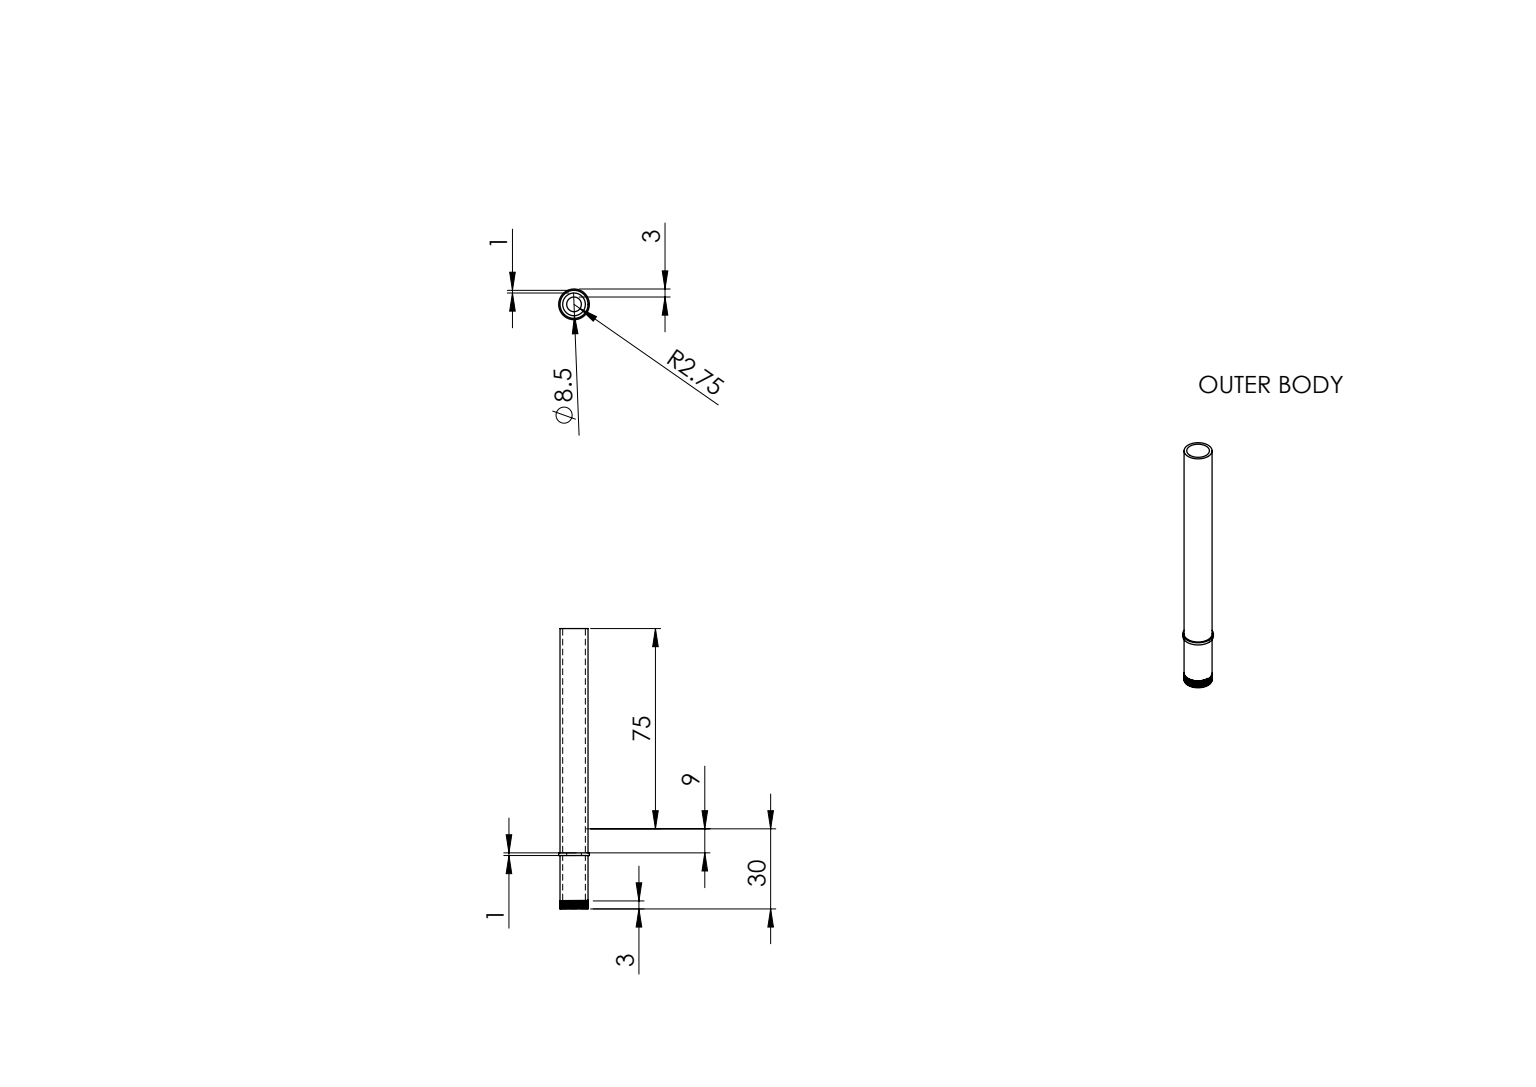
ISO-10303-21;
HEADER;
FILE_DESCRIPTION (('STEP AP214'),
    '1' );
FILE_NAME ('outer body.step',
    '2026-10-27T10:49:47',
    ( '' ),
    ( '' ),
    'SwSTEP 2.0',
    'SolidWorks 2026',
    '' );
FILE_SCHEMA (( 'AUTOMOTIVE_DESIGN' ));
ENDSEC;

DATA;
#4=CARTESIAN_POINT ( 'NONE',  ( 5.114683531250000748, -27.33854166700806587, -2.952963913586932776 ) ) ;
#6=CARTESIAN_POINT ( 'NONE',  ( 5.250000000000000000, -29.22916666666666430, -3.031088913245534755 ) ) ;
#8=ADVANCED_FACE ( 'NONE', ( #6134 ), #1014, .T. ) ;
#9=CARTESIAN_POINT ( 'NONE',  ( 5.114683531250000748, -28.90104166700806587, -2.952963913586932776 ) ) ;
#12=CARTESIAN_POINT ( 'NONE',  ( -5.114683531249999859, -28.31770833367473372, -2.952963913586935440 ) ) ;
#16=DIRECTION ( 'NONE',  ( 1.000000000000000000, 0.000000000000000000, -0.000000000000000000 ) ) ;
#17=CARTESIAN_POINT ( 'NONE',  ( -5.114683531249999859, -29.56770833367473017, -2.952963913586935440 ) ) ;
#19=EDGE_LOOP ( 'NONE', ( #3750, #4304, #1709, #1694 ) ) ;
#21=CARTESIAN_POINT ( 'NONE',  ( 2.557341765624996821, -29.15104166700806587, 4.429445870380401828 ) ) ;
#23=ORIENTED_EDGE ( 'NONE', *, *, #2711, .F. ) ;
#32=CARTESIAN_POINT ( 'NONE',  ( -5.114683531249999859, -28.75520833367473017, -2.952963913586935440 ) ) ;
#37=( BOUNDED_CURVE ( )  B_SPLINE_CURVE ( 2, ( #980, #8007, #3923, #3739, #4569, #5213, #3046, #6700, #6561 ),
 .UNSPECIFIED., .F., .F. ) 
 B_SPLINE_CURVE_WITH_KNOTS ( ( 3, 2, 2, 2, 3 ),
 ( 0.1041666666666666713, 0.1111111111111111049, 0.1250000000000000000, 0.1388888888888888951, 0.1458333333333333426 ),
 .UNSPECIFIED. ) 
 CURVE ( )  GEOMETRIC_REPRESENTATION_ITEM ( )  RATIONAL_B_SPLINE_CURVE ( ( 0.9330127018922194093, 0.9330127018922194093, 1.000000000000000000, 0.8660254037844387076, 1.000000000000000000, 0.8660254037844387076, 1.000000000000000000, 0.9330127018922194093, 0.9330127018922194093 ) ) 
 REPRESENTATION_ITEM ( '' )  );
#41=VECTOR ( 'NONE', #4397, 1000.000000000000000 ) ;
#44=CARTESIAN_POINT ( 'NONE',  ( 2.033577675846918216E-14, -27.81249999999999645, 5.250000000000000888 ) ) ;
#45=ORIENTED_EDGE ( 'NONE', *, *, #6013, .T. ) ;
#52=CARTESIAN_POINT ( 'NONE',  ( -2.624999999999998668, -28.91666666666666785, -4.546633369868303021 ) ) ;
#55=CARTESIAN_POINT ( 'NONE',  ( 5.114683531250000748, -28.42187500034139802, 0.000000000000000000 ) ) ;
#56=CARTESIAN_POINT ( 'NONE',  ( 3.616337804771879580E-16, -28.35937500034139447, -5.905927827173866440 ) ) ;
#65=CARTESIAN_POINT ( 'NONE',  ( 5.250000000000000000, -27.03125000068279604, 0.000000000000000000 ) ) ;
#74=EDGE_CURVE ( 'NONE', #2716, #8116, #2372, .T. ) ;
#76=CARTESIAN_POINT ( 'NONE',  ( -2.557341765624999042, -27.02604166700806232, -4.429445870380400052 ) ) ;
#79=EDGE_CURVE ( 'NONE', #7374, #1200, #6541, .T. ) ;
#83=FACE_OUTER_BOUND ( 'NONE', #879, .T. ) ;
#84=CARTESIAN_POINT ( 'NONE',  ( 0.000000000000000000, -30.00000000000000000, 0.000000000000000000 ) ) ;
#88=EDGE_LOOP ( 'NONE', ( #8020, #7590 ) ) ;
#91=ORIENTED_EDGE ( 'NONE', *, *, #709, .F. ) ;
#92=CARTESIAN_POINT ( 'NONE',  ( -2.625000000000002220, -28.58333333333333215, 4.546633369868302132 ) ) ;
#93=CYLINDRICAL_SURFACE ( 'NONE', #1391, 5.250000000000000000 ) ;
#94=CARTESIAN_POINT ( 'NONE',  ( -5.114683531250000748, -28.06770833367473017, -2.952963913586935440 ) ) ;
#96=CARTESIAN_POINT ( 'NONE',  ( 5.114683531249998971, -27.44270833367473017, 2.952963913586936329 ) ) ;
#100=CARTESIAN_POINT ( 'NONE',  ( 0.000000000000000000, -30.00000000000000000, 4.250000000000000000 ) ) ;
#102=CARTESIAN_POINT ( 'NONE',  ( -5.250000000000000888, -27.38541666734946389, 3.031088913245533423 ) ) ;
#103=CARTESIAN_POINT ( 'NONE',  ( 3.616337804771879580E-16, -29.60937500034139447, -5.905927827173866440 ) ) ;
#108=CARTESIAN_POINT ( 'NONE',  ( -2.557341765624999042, -28.27604166700806587, -4.429445870380400052 ) ) ;
#109=EDGE_LOOP ( 'NONE', ( #5447, #4357, #2145, #3993 ) ) ;
#111=ORIENTED_EDGE ( 'NONE', *, *, #9064, .F. ) ;
#118=CARTESIAN_POINT ( 'NONE',  ( 5.250000000000000000, -29.03125000068279604, 0.000000000000000000 ) ) ;
#121=CARTESIAN_POINT ( 'NONE',  ( 2.557341765624996821, -27.15104166700806587, 4.429445870380401828 ) ) ;
#124=CYLINDRICAL_SURFACE ( 'NONE', #4810, 5.250000000000000000 ) ;
#126=LINE ( 'NONE', #643, #8886 ) ;
#130=CARTESIAN_POINT ( 'NONE',  ( 0.000000000000000000, -9.999999999999998224, 0.000000000000000000 ) ) ;
#132=ORIENTED_EDGE ( 'NONE', *, *, #6059, .F. ) ;
#136=AXIS2_PLACEMENT_3D ( 'NONE', #8169, #1046, #2544 ) ;
#140=CARTESIAN_POINT ( 'NONE',  ( 2.624999999999996891, -29.04166666666666785, 4.546633369868304797 ) ) ;
#141=CARTESIAN_POINT ( 'NONE',  ( 2.624999999999996891, -29.79166666666666430, 4.546633369868304797 ) ) ;
#143=CARTESIAN_POINT ( 'NONE',  ( 5.114683531250000748, -27.67187500034139802, 0.000000000000000000 ) ) ;
#145=( LENGTH_UNIT ( ) NAMED_UNIT ( * ) SI_UNIT ( .MILLI., .METRE. ) );
#146=CARTESIAN_POINT ( 'NONE',  ( 3.616337804771879580E-16, -27.35937500034140157, -5.905927827173866440 ) ) ;
#148=DIRECTION ( 'NONE',  ( 0.000000000000000000, 0.000000000000000000, 1.000000000000000000 ) ) ;
#157=CARTESIAN_POINT ( 'NONE',  ( 2.557341765624996821, -28.65104166700806587, 4.429445870380401828 ) ) ;
#158=ORIENTED_EDGE ( 'NONE', *, *, #8454, .T. ) ;
#159=DIRECTION ( 'NONE',  ( 0.000000000000000000, 0.000000000000000000, 1.000000000000000000 ) ) ;
#163=ORIENTED_EDGE ( 'NONE', *, *, #1050, .T. ) ;
#165=CARTESIAN_POINT ( 'NONE',  ( 5.250000000000000000, -29.89062500034139802, 0.000000000000000000 ) ) ;
#168=CARTESIAN_POINT ( 'NONE',  ( 2.557341765625000818, -27.56770833367473017, -4.429445870380400052 ) ) ;
#186=VECTOR ( 'NONE', #298, 1000.000000000000000 ) ;
#188=CARTESIAN_POINT ( 'NONE',  ( -5.250000000000000000, -27.62500000000000000, -6.429395695523604153E-16 ) ) ;
#189=CARTESIAN_POINT ( 'NONE',  ( 3.616337804771879580E-16, -28.35937500034139447, -5.905927827173866440 ) ) ;
#191=EDGE_CURVE ( 'NONE', #7471, #2074, #636, .T. ) ;
#192=CARTESIAN_POINT ( 'NONE',  ( 2.557341765624996821, -26.96354166700806232, 4.429445870380401828 ) ) ;
#193=CARTESIAN_POINT ( 'NONE',  ( -1.084901341431563726E-15, -29.67187500034139802, 5.905927827173866440 ) ) ;
#197=VECTOR ( 'NONE', #5888, 1000.000000000000000 ) ;
#199=CARTESIAN_POINT ( 'NONE',  ( 5.114683531250000748, -29.67187500034139802, 0.000000000000000000 ) ) ;
#200=CARTESIAN_POINT ( 'NONE',  ( 2.624999999999996891, -27.32291666734946389, 4.546633369868304797 ) ) ;
#202=ORIENTED_EDGE ( 'NONE', *, *, #7606, .T. ) ;
#205=CARTESIAN_POINT ( 'NONE',  ( 3.616337804771879580E-16, -28.04687500034139802, -5.905927827173866440 ) ) ;
#214=CARTESIAN_POINT ( 'NONE',  ( -1.113604000661152470E-15, -29.09375000068279249, 6.062177826491070398 ) ) ;
#216=CARTESIAN_POINT ( 'NONE',  ( -5.114683531249999859, -27.50520833367472662, -2.952963913586935440 ) ) ;
#217=CARTESIAN_POINT ( 'NONE',  ( 0.000000000000000000, -9.000000000000000000, 0.000000000000000000 ) ) ;
#218=FACE_OUTER_BOUND ( 'NONE', #2298, .T. ) ;
#222=EDGE_CURVE ( 'NONE', #8837, #8220, #2702, .T. ) ;
#235=ORIENTED_EDGE ( 'NONE', *, *, #430, .T. ) ;
#236=CARTESIAN_POINT ( 'NONE',  ( 5.250000000000000000, -27.22916666666666430, -3.031088913245534755 ) ) ;
#237=CARTESIAN_POINT ( 'NONE',  ( -5.114683531250000748, -28.31770833367473728, -2.952963913586935440 ) ) ;
#239=DIRECTION ( 'NONE',  ( -0.000000000000000000, 1.000000000000000000, -0.000000000000000000 ) ) ;
#242=CARTESIAN_POINT ( 'NONE',  ( -5.114683531250000748, -28.27604166700806232, 2.952963913586931888 ) ) ;
#245=CARTESIAN_POINT ( 'NONE',  ( 6.972266317189433020E-16, -29.43750000000000000, -5.250000000000000000 ) ) ;
#246=CARTESIAN_POINT ( 'NONE',  ( 2.557341765625000818, -28.31770833367473017, -4.429445870380400052 ) ) ;
#256=CARTESIAN_POINT ( 'NONE',  ( 5.250000000000000000, -29.51041666734946034, -3.031088913245534755 ) ) ;
#259=CARTESIAN_POINT ( 'NONE',  ( -1.084901341431563923E-15, -27.17187500034140157, 5.905927827173866440 ) ) ;
#260=ORIENTED_EDGE ( 'NONE', *, *, #6679, .T. ) ;
#273=CARTESIAN_POINT ( 'NONE',  ( -1.406733260263395735, -29.57366454968462932, 5.250000000000000000 ) ) ;
#274=ORIENTED_EDGE ( 'NONE', *, *, #6013, .F. ) ;
#278=CARTESIAN_POINT ( 'NONE',  ( -5.250000000000000000, -27.87500000000000000, -6.429395695523604153E-16 ) ) ;
#283=CARTESIAN_POINT ( 'NONE',  ( -2.557341765625002594, -27.00520833367473017, 4.429445870380399164 ) ) ;
#284=CARTESIAN_POINT ( 'NONE',  ( 3.616337804771879580E-16, -28.79687500034140157, -5.905927827173866440 ) ) ;
#287=CARTESIAN_POINT ( 'NONE',  ( 0.000000000000000000, -30.00000000000000000, 4.250000000000000000 ) ) ;
#288=CARTESIAN_POINT ( 'NONE',  ( 2.557341765624996821, -29.21354166700806587, 4.429445870380401828 ) ) ;
#289=CARTESIAN_POINT ( 'NONE',  ( -1.975475456537005874E-15, -27.34375000068279249, 5.250000000000000000 ) ) ;
#293=CARTESIAN_POINT ( 'NONE',  ( -1.406733260263395735, -29.32366454968462932, 5.250000000000000000 ) ) ;
#294=CARTESIAN_POINT ( 'NONE',  ( 5.114683531249999859, -29.08854166700806942, -2.952963913586932776 ) ) ;
#298=DIRECTION ( 'NONE',  ( 0.000000000000000000, 1.000000000000000000, 0.000000000000000000 ) ) ;
#304=CARTESIAN_POINT ( 'NONE',  ( -5.250000000000000000, -29.40625000068279604, -6.429395695523604153E-16 ) ) ;
#308=CARTESIAN_POINT ( 'NONE',  ( 0.000000000000000000, -30.00000000000000000, 0.000000000000000000 ) ) ;
#312=CARTESIAN_POINT ( 'NONE',  ( 0.000000000000000000, -9.000000000000001776, 4.250000000000000000 ) ) ;
#324=CARTESIAN_POINT ( 'NONE',  ( -1.113604000661152470E-15, -28.06249999999999645, 6.062177826491070398 ) ) ;
#325=CARTESIAN_POINT ( 'NONE',  ( 5.114683531250000748, -26.92187500034139802, 0.000000000000000000 ) ) ;
#330=CARTESIAN_POINT ( 'NONE',  ( -5.114683531250001636, -29.46354166700806232, 2.952963913586931444 ) ) ;
#331=( BOUNDED_CURVE ( )  B_SPLINE_CURVE ( 2, ( #289, #2486, #200, #3691, #3189, #5309, #5871, #6202, #3416 ),
 .UNSPECIFIED., .F., .F. ) 
 B_SPLINE_CURVE_WITH_KNOTS ( ( 3, 2, 2, 2, 3 ),
 ( 0.8125000000000000000, 0.8194444444444444198, 0.8333333333333333703, 0.8472222222222222099, 0.8541666666666666297 ),
 .UNSPECIFIED. ) 
 CURVE ( )  GEOMETRIC_REPRESENTATION_ITEM ( )  RATIONAL_B_SPLINE_CURVE ( ( 0.9330127018922194093, 0.9330127018922194093, 1.000000000000000000, 0.8660254037844387076, 1.000000000000000000, 0.8660254037844387076, 1.000000000000000000, 0.9330127018922198534, 0.9330127018922192983 ) ) 
 REPRESENTATION_ITEM ( '' )  );
#333=CARTESIAN_POINT ( 'NONE',  ( 6.972266317189433020E-16, -28.46875000068279959, -5.250000000000000000 ) ) ;
#335=CARTESIAN_POINT ( 'NONE',  ( 2.557341765625000818, -28.38020833367473017, -4.429445870380400052 ) ) ;
#336=AXIS2_PLACEMENT_3D ( 'NONE', #5769, #2196, #6511 ) ;
#338=CARTESIAN_POINT ( 'NONE',  ( 5.114683531250000748, -29.90104166700806232, -2.952963913586932776 ) ) ;
#339=EDGE_LOOP ( 'NONE', ( #7797, #3924, #3008, #7248 ) ) ;
#345=UNCERTAINTY_MEASURE_WITH_UNIT (LENGTH_MEASURE( 1.000000000000000082E-05 ), #5708, 'distance_accuracy_value', 'NONE');
#346=DIRECTION ( 'NONE',  ( 0.000000000000000000, 1.000000000000000000, 0.000000000000000000 ) ) ;
#351=CARTESIAN_POINT ( 'NONE',  ( -2.624999999999998668, -27.94791666734946389, -4.546633369868303021 ) ) ;
#353=ORIENTED_EDGE ( 'NONE', *, *, #8523, .F. ) ;
#356=CARTESIAN_POINT ( 'NONE',  ( 0.000000000000000000, -30.00000000000000000, 0.000000000000000000 ) ) ;
#357=PRODUCT_DEFINITION_SHAPE ( 'NONE', 'NONE',  #9105 ) ;
#358=EDGE_CURVE ( 'NONE', #6742, #3365, #4804, .T. ) ;
#362=EDGE_CURVE ( 'NONE', #849, #3341, #1779, .T. ) ;
#363=CARTESIAN_POINT ( 'NONE',  ( 1.406733260263402174, -27.80133545031536713, 5.249999999999995559 ) ) ;
#367=EDGE_CURVE ( 'NONE', #5103, #6258, #7983, .T. ) ;
#373=CARTESIAN_POINT ( 'NONE',  ( 3.712013335537174572E-16, -27.93749999999999645, -6.062177826491070398 ) ) ;
#375=CARTESIAN_POINT ( 'NONE',  ( -5.114683531250000748, -27.06770833367473017, -2.952963913586935440 ) ) ;
#376=ORIENTED_EDGE ( 'NONE', *, *, #4348, .F. ) ;
#378=EDGE_LOOP ( 'NONE', ( #5714, #6318, #4777, #2554 ) ) ;
#379=CARTESIAN_POINT ( 'NONE',  ( 5.114683531249998971, -29.63020833367473017, 2.952963913586936329 ) ) ;
#382=CARTESIAN_POINT ( 'NONE',  ( -1.406733260263382856, -28.17633545031537068, -5.250000000000006217 ) ) ;
#383=CARTESIAN_POINT ( 'NONE',  ( 3.616337804771879580E-16, -28.85937500034139802, -5.905927827173866440 ) ) ;
#385=CARTESIAN_POINT ( 'NONE',  ( -5.250000000000000000, -27.90625000068279604, -6.429395695523604153E-16 ) ) ;
#386=CARTESIAN_POINT ( 'NONE',  ( -2.557341765624999042, -27.02604166700806232, -4.429445870380400052 ) ) ;
#392=CARTESIAN_POINT ( 'NONE',  ( -1.406733260263395735, -29.10491455036742536, 5.250000000000000000 ) ) ;
#393=CARTESIAN_POINT ( 'NONE',  ( 2.625000000000000444, -29.95833333333333215, -4.546633369868303021 ) ) ;
#398=CARTESIAN_POINT ( 'NONE',  ( -2.625000000000002220, -28.36458333401612819, 4.546633369868302132 ) ) ;
#403=CARTESIAN_POINT ( 'NONE',  ( 2.624999999999996891, -29.54166666666666430, 4.546633369868304797 ) ) ;
#405=DIRECTION ( 'NONE',  ( -1.000000000000000000, 0.000000000000000000, -0.000000000000000000 ) ) ;
#406=CARTESIAN_POINT ( 'NONE',  ( 5.114683531250000748, -26.85937500034139802, 0.000000000000000000 ) ) ;
#407=CARTESIAN_POINT ( 'NONE',  ( 2.557341765624996821, -29.65104166700806232, 4.429445870380401828 ) ) ;
#412=CARTESIAN_POINT ( 'NONE',  ( 5.250000000000000000, -26.89062500034139802, 0.000000000000000000 ) ) ;
#416=CARTESIAN_POINT ( 'NONE',  ( 2.300847884672513123E-14, -27.21875000068279959, -5.250000000000000000 ) ) ;
#418=LINE ( 'NONE', #4145, #7439 ) ;
#419=ADVANCED_FACE ( 'NONE', ( #7237, #2173 ), #774, .T. ) ;
#424=AXIS2_PLACEMENT_3D ( 'NONE', #4231, #5705, #777 ) ;
#425=CARTESIAN_POINT ( 'NONE',  ( 5.114683531250000748, -28.85937500034139802, 0.000000000000000000 ) ) ;
#428=CARTESIAN_POINT ( 'NONE',  ( -5.114683531250000748, -29.02604166700806587, 2.952963913586931888 ) ) ;
#430=EDGE_CURVE ( 'NONE', #3312, #7207, #3019, .T. ) ;
#431=CARTESIAN_POINT ( 'NONE',  ( -2.624999999999998668, -27.94791666734946389, -4.546633369868303021 ) ) ;
#432=CARTESIAN_POINT ( 'NONE',  ( 0.000000000000000000, -30.00000000000000000, 0.000000000000000000 ) ) ;
#433=AXIS2_PLACEMENT_3D ( 'NONE', #4506, #7382, #7240 ) ;
#434=CARTESIAN_POINT ( 'NONE',  ( -1.406733260263395735, -28.32366454968462577, 5.250000000000000000 ) ) ;
#436=CARTESIAN_POINT ( 'NONE',  ( 5.114683531250000748, -29.67187500034139802, 0.000000000000000000 ) ) ;
#440=CARTESIAN_POINT ( 'NONE',  ( 9.180150650966086169E-15, -28.56249999999999645, 5.250000000000000000 ) ) ;
#441=LINE ( 'NONE', #9040, #870 ) ;
#447=DIRECTION ( 'NONE',  ( -0.000000000000000000, -1.000000000000000000, -0.000000000000000000 ) ) ;
#448=CARTESIAN_POINT ( 'NONE',  ( -5.250000000000000000, -27.92708333401612819, -3.031088913245536531 ) ) ;
#459=CARTESIAN_POINT ( 'NONE',  ( 2.557341765625000818, -29.31770833367473017, -4.429445870380400052 ) ) ;
#460=ORIENTED_EDGE ( 'NONE', *, *, #7717, .T. ) ;
#467=VECTOR ( 'NONE', #3569, 1000.000000000000000 ) ;
#472=ORIENTED_EDGE ( 'NONE', *, *, #8246, .T. ) ;
#476=CARTESIAN_POINT ( 'NONE',  ( -5.114683531250001636, -29.21354166700806587, 2.952963913586931444 ) ) ;
#478=FACE_OUTER_BOUND ( 'NONE', #6239, .T. ) ;
#479=CARTESIAN_POINT ( 'NONE',  ( -5.114683531250000748, -27.79687500034139802, -6.263680815196995234E-16 ) ) ;
#482=CARTESIAN_POINT ( 'NONE',  ( 2.300847884672513123E-14, -27.96875000068279959, -5.250000000000000000 ) ) ;
#483=DIRECTION ( 'NONE',  ( 0.000000000000000000, 1.000000000000000000, 0.000000000000000000 ) ) ;
#484=CARTESIAN_POINT ( 'NONE',  ( 0.000000000000000000, -30.00000000000000000, 0.000000000000000000 ) ) ;
#485=CARTESIAN_POINT ( 'NONE',  ( -2.557341765624999042, -29.58854166700806232, -4.429445870380400052 ) ) ;
#490=CARTESIAN_POINT ( 'NONE',  ( 0.000000000000000000, -9.999999999999998224, 0.000000000000000000 ) ) ;
#494=VECTOR ( 'NONE', #3689, 1000.000000000000000 ) ;
#495=ORIENTED_EDGE ( 'NONE', *, *, #3861, .T. ) ;
#497=CARTESIAN_POINT ( 'NONE',  ( 2.625000000000000444, -29.23958333401613174, -4.546633369868303021 ) ) ;
#498=CARTESIAN_POINT ( 'NONE',  ( 5.250000000000000000, -27.78125000068279604, 0.000000000000000000 ) ) ;
#500=AXIS2_PLACEMENT_3D ( 'NONE', #4103, #6277, #6092 ) ;
#505=CARTESIAN_POINT ( 'NONE',  ( 2.625000000000000444, -29.73958333401613174, -4.546633369868303021 ) ) ;
#508=DIRECTION ( 'NONE',  ( 0.000000000000000000, 1.000000000000000000, 0.000000000000000000 ) ) ;
#510=FACE_OUTER_BOUND ( 'NONE', #109, .T. ) ;
#513=EDGE_CURVE ( 'NONE', #1200, #7933, #6888, .T. ) ;
#517=EDGE_CURVE ( 'NONE', #2565, #5103, #5524, .T. ) ;
#519=EDGE_LOOP ( 'NONE', ( #1240, #6626, #8877, #4519 ) ) ;
#525=APPLICATION_CONTEXT ( 'automotive_design' ) ;
#526=CARTESIAN_POINT ( 'NONE',  ( -1.084901341431563726E-15, -27.42187500034139802, 5.905927827173866440 ) ) ;
#528=DIRECTION ( 'NONE',  ( 0.000000000000000000, 0.000000000000000000, 1.000000000000000000 ) ) ;
#529=CARTESIAN_POINT ( 'NONE',  ( 5.114683531249998971, -27.44270833367473017, 2.952963913586936329 ) ) ;
#532=CARTESIAN_POINT ( 'NONE',  ( 3.616337804771879580E-16, -29.60937500034139447, -5.905927827173866440 ) ) ;
#534=CARTESIAN_POINT ( 'NONE',  ( -5.114683531250000748, -28.54687500034139802, -6.263680815196995234E-16 ) ) ;
#541=ORIENTED_EDGE ( 'NONE', *, *, #4558, .F. ) ;
#544=CARTESIAN_POINT ( 'NONE',  ( -1.113604000661152470E-15, -28.34375000068279249, 6.062177826491070398 ) ) ;
#547=ORIENTED_EDGE ( 'NONE', *, *, #6137, .F. ) ;
#550=CARTESIAN_POINT ( 'NONE',  ( 5.250000000000000000, -29.50000000000000000, 0.000000000000000000 ) ) ;
#553=ADVANCED_FACE ( 'NONE', ( #4389 ), #8133, .T. ) ;
#555=CARTESIAN_POINT ( 'NONE',  ( -1.084901341431563923E-15, -29.67187500034139802, 5.905927827173866440 ) ) ;
#556=CARTESIAN_POINT ( 'NONE',  ( 1.406733260263402174, -27.58258545099816317, 5.249999999999995559 ) ) ;
#560=CYLINDRICAL_SURFACE ( 'NONE', #5921, 5.250000000000000000 ) ;
#564=CYLINDRICAL_SURFACE ( 'NONE', #5351, 5.250000000000000000 ) ;
#566=VERTEX_POINT ( 'NONE', #5578 ) ;
#568=CARTESIAN_POINT ( 'NONE',  ( -1.084901341431563726E-15, -28.17187500034139447, 5.905927827173866440 ) ) ;
#571=CARTESIAN_POINT ( 'NONE',  ( -5.250000000000000000, -29.89583333333333215, -3.031088913245536531 ) ) ;
#573=CARTESIAN_POINT ( 'NONE',  ( -5.114683531250001636, -28.77604166700806587, 2.952963913586931444 ) ) ;
#575=AXIS2_PLACEMENT_3D ( 'NONE', #8304, #7511, #3982 ) ;
#576=CARTESIAN_POINT ( 'NONE',  ( -5.114683531250000748, -29.52604166700806232, 2.952963913586931888 ) ) ;
#588=CARTESIAN_POINT ( 'NONE',  ( -1.113604000661152470E-15, -27.34375000068279959, 6.062177826491070398 ) ) ;
#598=CARTESIAN_POINT ( 'NONE',  ( 3.616337804771879580E-16, -29.04687500034139802, -5.905927827173866440 ) ) ;
#603=LINE ( 'NONE', #412, #1926 ) ;
#608=CYLINDRICAL_SURFACE ( 'NONE', #8342, 5.250000000000000000 ) ;
#609=EDGE_CURVE ( 'NONE', #3341, #6499, #9020, .T. ) ;
#613=CARTESIAN_POINT ( 'NONE',  ( -1.084901341431563726E-15, -27.17187500034139802, 5.905927827173866440 ) ) ;
#615=CARTESIAN_POINT ( 'NONE',  ( 2.557341765625000818, -27.38020833367473017, -4.429445870380400052 ) ) ;
#616=DIRECTION ( 'NONE',  ( 0.000000000000000000, 1.000000000000000000, 0.000000000000000000 ) ) ;
#617=CARTESIAN_POINT ( 'NONE',  ( -5.114683531250000748, -29.56770833367472662, -2.952963913586935440 ) ) ;
#619=CARTESIAN_POINT ( 'NONE',  ( -1.084901341431563923E-15, -28.73437500034139802, 5.905927827173866440 ) ) ;
#620=CARTESIAN_POINT ( 'NONE',  ( -2.624999999999998668, -29.66666666666666430, -4.546633369868303021 ) ) ;
#627=VERTEX_POINT ( 'NONE', #4875 ) ;
#629=CARTESIAN_POINT ( 'NONE',  ( 3.712013335537174572E-16, -26.96875000068279249, -6.062177826491070398 ) ) ;
#636=CIRCLE ( 'NONE', #3913, 5.250000000000000000 ) ;
#638=CARTESIAN_POINT ( 'NONE',  ( 6.972266317189433020E-16, -27.71875000068279604, -5.250000000000000000 ) ) ;
#639=CARTESIAN_POINT ( 'NONE',  ( 5.114683531249999859, -28.83854166700806587, -2.952963913586932776 ) ) ;
#640=CARTESIAN_POINT ( 'NONE',  ( 0.000000000000000000, -9.000000000000001776, 0.000000000000000000 ) ) ;
#643=CARTESIAN_POINT ( 'NONE',  ( 7.041719095097280880E-16, -9.999999999999998224, -5.750000000000000000 ) ) ;
#657=CARTESIAN_POINT ( 'NONE',  ( 3.616337804771879580E-16, -28.04687500034139802, -5.905927827173866440 ) ) ;
#659=CARTESIAN_POINT ( 'NONE',  ( 5.114683531250000748, -27.17187500034139802, 0.000000000000000000 ) ) ;
#661=CARTESIAN_POINT ( 'NONE',  ( 5.114683531250000748, -28.92187500034139802, 0.000000000000000000 ) ) ;
#662=CARTESIAN_POINT ( 'NONE',  ( 5.114683531250000748, -28.17187500034139447, 0.000000000000000000 ) ) ;
#669=ORIENTED_EDGE ( 'NONE', *, *, #756, .T. ) ;
#671=CARTESIAN_POINT ( 'NONE',  ( 3.616337804771879580E-16, -29.29687500034139447, -5.905927827173866440 ) ) ;
#672=EDGE_CURVE ( 'NONE', #8760, #977, #1244, .T. ) ;
#676=PLANE ( 'NONE',  #2520 ) ;
#680=CARTESIAN_POINT ( 'NONE',  ( 1.406733260263394625, -27.72991455036742536, -5.250000000000000000 ) ) ;
#681=CARTESIAN_POINT ( 'NONE',  ( -5.114683531250000748, -28.71354166700806587, 2.952963913586931888 ) ) ;
#683=CARTESIAN_POINT ( 'NONE',  ( -5.249999999999999112, -28.92708333401613174, -3.031088913245536975 ) ) ;
#692=ORIENTED_EDGE ( 'NONE', *, *, #6725, .T. ) ;
#695=CARTESIAN_POINT ( 'NONE',  ( -5.114683531250001636, -28.21354166700806587, 2.952963913586931444 ) ) ;
#697=CARTESIAN_POINT ( 'NONE',  ( 5.250000000000000000, -29.72916666666666430, -3.031088913245534755 ) ) ;
#698=EDGE_CURVE ( 'NONE', #4680, #6430, #9079, .T. ) ;
#700=CARTESIAN_POINT ( 'NONE',  ( 3.616337804771879580E-16, -29.85937500034140157, -5.905927827173866440 ) ) ;
#701=CARTESIAN_POINT ( 'NONE',  ( -2.557341765624999042, -27.58854166700806587, -4.429445870380400052 ) ) ;
#709=EDGE_CURVE ( 'NONE', #2565, #1880, #9113, .T. ) ;
#710=ORIENTED_EDGE ( 'NONE', *, *, #1444, .T. ) ;
#712=CARTESIAN_POINT ( 'NONE',  ( -5.250000000000000000, -27.17708333401612819, -3.031088913245536531 ) ) ;
#714=ORIENTED_EDGE ( 'NONE', *, *, #709, .T. ) ;
#725=CARTESIAN_POINT ( 'NONE',  ( 2.557341765624996821, -28.90104166700806587, 4.429445870380401828 ) ) ;
#727=CARTESIAN_POINT ( 'NONE',  ( 1.185285273922203525E-14, -28.96875000068279959, -5.250000000000000000 ) ) ;
#729=CARTESIAN_POINT ( 'NONE',  ( 5.204748896376250699E-16, -9.000000000000001776, -4.250000000000000000 ) ) ;
#732=VECTOR ( 'NONE', #6064, 1000.000000000000000 ) ;
#733=DIRECTION ( 'NONE',  ( -0.000000000000000000, -1.000000000000000000, -0.000000000000000000 ) ) ;
#744=CARTESIAN_POINT ( 'NONE',  ( -1.113604000661152470E-15, -29.81250000000000000, 6.062177826491070398 ) ) ;
#745=DIRECTION ( 'NONE',  ( 0.000000000000000000, 0.000000000000000000, 1.000000000000000000 ) ) ;
#746=CARTESIAN_POINT ( 'NONE',  ( -2.557341765625002594, -28.50520833367473017, 4.429445870380399164 ) ) ;
#749=CARTESIAN_POINT ( 'NONE',  ( -2.557341765624999042, -28.08854166700806587, -4.429445870380400052 ) ) ;
#752=CARTESIAN_POINT ( 'NONE',  ( 5.249999999999997335, -29.55208333401613885, 3.031088913245538308 ) ) ;
#753=CARTESIAN_POINT ( 'NONE',  ( 2.300847884672513123E-14, -28.43750000000000000, -5.250000000000000000 ) ) ;
#754=CARTESIAN_POINT ( 'NONE',  ( 5.114683531249998971, -29.44270833367473372, 2.952963913586936329 ) ) ;
#756=EDGE_CURVE ( 'NONE', #7705, #8808, #3387, .T. ) ;
#760=CARTESIAN_POINT ( 'NONE',  ( -1.084901341431563923E-15, -29.67187500034139802, 5.905927827173866440 ) ) ;
#763=( BOUNDED_CURVE ( )  B_SPLINE_CURVE ( 2, ( #6831, #8182, #8914, #7483, #3951, #7577, #6926, #6129, #8961 ),
 .UNSPECIFIED., .F., .T. ) 
 B_SPLINE_CURVE_WITH_KNOTS ( ( 3, 2, 2, 2, 3 ),
 ( 0.3541666666666666297, 0.3611111111111111049, 0.3750000000000000000, 0.3888888888888888951, 0.3958333333333333703 ),
 .UNSPECIFIED. ) 
 CURVE ( )  GEOMETRIC_REPRESENTATION_ITEM ( )  RATIONAL_B_SPLINE_CURVE ( ( 0.9330127018922194093, 0.9330127018922190762, 1.000000000000000000, 0.8660254037844387076, 1.000000000000000000, 0.8660254037844387076, 1.000000000000000000, 0.9330127018922190762, 0.9330127018922194093 ) ) 
 REPRESENTATION_ITEM ( '' )  );
#773=CARTESIAN_POINT ( 'NONE',  ( 5.114683531249999859, -28.58854166700806232, -2.952963913586932776 ) ) ;
#774=PLANE ( 'NONE',  #1388 ) ;
#775=CARTESIAN_POINT ( 'NONE',  ( 2.625000000000000444, -28.98958333401613174, -4.546633369868303021 ) ) ;
#777=DIRECTION ( 'NONE',  ( 0.000000000000000000, 0.000000000000000000, 1.000000000000000000 ) ) ;
#782=CARTESIAN_POINT ( 'NONE',  ( 6.972266317189433020E-16, -27.71875000068279604, -5.250000000000000000 ) ) ;
#784=VERTEX_POINT ( 'NONE', #5850 ) ;
#789=CARTESIAN_POINT ( 'NONE',  ( 0.000000000000000000, 75.00000000000000000, 5.250000000000000000 ) ) ;
#792=CARTESIAN_POINT ( 'NONE',  ( -5.250000000000000000, -28.64583333333332860, -3.031088913245536531 ) ) ;
#793=LINE ( 'NONE', #3457, #2596 ) ;
#794=CIRCLE ( 'NONE', #5842, 5.750000000000000000 ) ;
#795=CARTESIAN_POINT ( 'NONE',  ( 5.114683531250000748, -27.42187500034139802, 0.000000000000000000 ) ) ;
#796=CARTESIAN_POINT ( 'NONE',  ( -2.557341765625002594, -27.50520833367473017, 4.429445870380399164 ) ) ;
#798=CARTESIAN_POINT ( 'NONE',  ( -1.975475456537005874E-15, -29.59375000068279249, 5.249999999999999112 ) ) ;
#799=DIRECTION ( 'NONE',  ( 0.000000000000000000, 1.000000000000000000, 0.000000000000000000 ) ) ;
#801=CARTESIAN_POINT ( 'NONE',  ( -5.114683531250000748, -29.77604166700806232, 2.952963913586931888 ) ) ;
#803=VERTEX_POINT ( 'NONE', #1062 ) ;
#806=CARTESIAN_POINT ( 'NONE',  ( 5.114683531249999859, -27.83854166700806587, -2.952963913586932776 ) ) ;
#810=LINE ( 'NONE', #5926, #186 ) ;
#813=VERTEX_POINT ( 'NONE', #6729 ) ;
#815=CARTESIAN_POINT ( 'NONE',  ( -1.975475456537005874E-15, -29.34375000068279249, 5.250000000000000000 ) ) ;
#816=CARTESIAN_POINT ( 'NONE',  ( -5.250000000000000000, -29.42708333401613174, -3.031088913245536531 ) ) ;
#817=( BOUNDED_SURFACE ( )  B_SPLINE_SURFACE ( 1, 2, ( 
 ( #3707, #7233, #6674, #2454, #3848, #5280, #6532, #7376, #858, #2968, #5840, #8125, #5090, #256, #4446, #2262, #8679, #816, #304, #3157, #5137, #7284, #1562, #4359, #3108, #4403, #7192, #3757, #3657, #2403, #6585, #5932, #2356, #214, #4499, #6483, #118, #5185, #3066, #8773, #5791, #8633, #5885, #8723, #956, #1658, #8028, #7331, #5232, #8077, #1706, #6629, #4544, #8998, #1196, #3898, #3343, #1945, #2646, #6717, #8222, #1242, #4040, #5518, #7427, #6872, #6821, #3991, #398, #544, #1855, #6172, #4084, #5372, #3245, #6069, #2551, #2498, #7519, #7617, #3385, #1148, #8314, #8859, #6770, #1052, #4682, #5322, #351, #448, #1754, #6919, #7473, #8905, #3294, #4773, #498, #6217, #9046, #3201, #6122, #4590, #8951, #5467, #2691, #6022, #8176, #1899, #2602, #5419, #1802, #4635, #1103, #3943, #8268, #4726, #7568, #588, #3516, #4255, #3604, #1284, #5560, #7089, #2116, #712, #7799, #4215, #8361, #2735, #8446, #6429, #65, #4301, #6300, #629, #5601, #2162, #9137, #3472, #4899, #7662, #6957, #1456, #9092 ),
 ( #8534, #3432, #4818, #7751, #3560, #8495, #9176, #2781, #2915, #760, #7139, #4982, #6383, #4855, #2071, #1415, #1987, #8405, #4123, #6261, #2032, #7838, #6340, #7004, #7701, #5689, #1327, #671, #4170, #1373, #7047, #2826, #5646, #4941, #21, #2869, #6522, #294, #5223, #2301, #3749, #7223, #948, #3007, #1597, #7972, #4394, #1504, #8018, #848, #1553, #3098, #3696, #5028, #8714, #2394, #5076, #3649, #157, #1650, #3795, #8669, #4535, #2958, #4488, #5732, #5830, #990, #5125, #6619, #7321, #7930, #4437, #7273, #246, #5920, #108, #5779, #900, #6571, #3836, #8066, #8763, #6662, #8577, #1696, #7366, #205, #3056, #8622, #5876, #2205, #2345, #2252, #7885, #4347, #7183, #806, #5175, #6473, #8850, #1743, #6012, #1229, #3889, #8257, #3235, #1037, #2489, #8807, #8986, #2634, #3933, #4624, #4760, #7555, #3280, #2589, #3978, #5312, #8208, #1842, #1138, #1792, #1091, #2444, #1932, #6760, #4580, #1181, #5407, #5269, #4715, #3328, #4025, #8115, #386, #5455, #1890, #6907, #7415, #6860, #4671, #5361, #7464 ) ),
 .UNSPECIFIED., .F., .F., .F. ) 
 B_SPLINE_SURFACE_WITH_KNOTS ( ( 2, 2 ),
 ( 3, 2, 2, 2, 2, 2, 2, 2, 2, 2, 2, 2, 2, 2, 2, 2, 2, 2, 2, 2, 2, 2, 2, 2, 2, 2, 2, 2, 2, 2, 2, 2, 2, 2, 2, 2, 2, 2, 2, 2, 2, 2, 2, 2, 2, 2, 2, 2, 2, 2, 2, 2, 2, 2, 2, 2, 2, 2, 2, 2, 2, 2, 2, 2, 2, 2, 2, 2, 2, 2, 2, 2, 3 ),
 ( 0.000000000000000000, 1.000000000000000000 ),
 ( 0.000000000000000000, 0.01388888888888888812, 0.02777777777777777624, 0.04166666666666666435, 0.05555555555555555247, 0.06944444444444444753, 0.08333333333333332871, 0.09722222222222222376, 0.1111111111111111049, 0.1250000000000000000, 0.1388888888888888951, 0.1527777777777777901, 0.1666666666666666574, 0.1805555555555555525, 0.1944444444444444475, 0.2083333333333333426, 0.2222222222222222099, 0.2361111111111111049, 0.2500000000000000000, 0.2638888888888888951, 0.2777777777777777901, 0.2916666666666666852, 0.3055555555555555802, 0.3194444444444444198, 0.3333333333333333148, 0.3472222222222222099, 0.3611111111111111049, 0.3750000000000000000, 0.3888888888888888951, 0.4027777777777777901, 0.4166666666666666852, 0.4305555555555555802, 0.4444444444444444198, 0.4583333333333333148, 0.4722222222222222099, 0.4861111111111111049, 0.5000000000000000000, 0.5138888888888888395, 0.5277777777777777901, 0.5416666666666666297, 0.5555555555555555802, 0.5694444444444444198, 0.5833333333333333703, 0.5972222222222222099, 0.6111111111111111605, 0.6250000000000000000, 0.6388888888888888395, 0.6527777777777777901, 0.6666666666666666297, 0.6805555555555555802, 0.6944444444444444198, 0.7083333333333333703, 0.7222222222222222099, 0.7361111111111111605, 0.7500000000000000000, 0.7638888888888888395, 0.7777777777777777901, 0.7916666666666666297, 0.8055555555555555802, 0.8194444444444444198, 0.8333333333333333703, 0.8472222222222222099, 0.8611111111111111605, 0.8750000000000000000, 0.8888888888888888395, 0.9027777777777777901, 0.9166666666666666297, 0.9305555555555555802, 0.9444444444444444198, 0.9583333333333333703, 0.9722222222222222099, 0.9861111111111111605, 1.000000000000000000 ),
 .UNSPECIFIED. ) 
 GEOMETRIC_REPRESENTATION_ITEM ( )  RATIONAL_B_SPLINE_SURFACE ( (
 ( 1.000000000000000000, 0.8660254037844387076, 1.000000000000000000, 0.8660254037844387076, 1.000000000000000000, 0.8660254037844387076, 1.000000000000000000, 0.8660254037844387076, 1.000000000000000000, 0.8660254037844387076, 1.000000000000000000, 0.8660254037844387076, 1.000000000000000000, 0.8660254037844387076, 1.000000000000000000, 0.8660254037844387076, 1.000000000000000000, 0.8660254037844387076, 1.000000000000000000, 0.8660254037844387076, 1.000000000000000000, 0.8660254037844387076, 1.000000000000000000, 0.8660254037844387076, 1.000000000000000000, 0.8660254037844387076, 1.000000000000000000, 0.8660254037844387076, 1.000000000000000000, 0.8660254037844387076, 1.000000000000000000, 0.8660254037844387076, 1.000000000000000000, 0.8660254037844387076, 1.000000000000000000, 0.8660254037844387076, 1.000000000000000000, 0.8660254037844387076, 1.000000000000000000, 0.8660254037844387076, 1.000000000000000000, 0.8660254037844387076, 1.000000000000000000, 0.8660254037844387076, 1.000000000000000000, 0.8660254037844387076, 1.000000000000000000, 0.8660254037844387076, 1.000000000000000000, 0.8660254037844387076, 1.000000000000000000, 0.8660254037844387076, 1.000000000000000000, 0.8660254037844387076, 1.000000000000000000, 0.8660254037844387076, 1.000000000000000000, 0.8660254037844387076, 1.000000000000000000, 0.8660254037844387076, 1.000000000000000000, 0.8660254037844387076, 1.000000000000000000, 0.8660254037844387076, 1.000000000000000000, 0.8660254037844387076, 1.000000000000000000, 0.8660254037844387076, 1.000000000000000000, 0.8660254037844387076, 1.000000000000000000, 0.8660254037844387076, 1.000000000000000000, 0.8660254037844387076, 1.000000000000000000, 0.8660254037844387076, 1.000000000000000000, 0.8660254037844387076, 1.000000000000000000, 0.8660254037844387076, 1.000000000000000000, 0.8660254037844387076, 1.000000000000000000, 0.8660254037844387076, 1.000000000000000000, 0.8660254037844387076, 1.000000000000000000, 0.8660254037844387076, 1.000000000000000000, 0.8660254037844387076, 1.000000000000000000, 0.8660254037844387076, 1.000000000000000000, 0.8660254037844387076, 1.000000000000000000, 0.8660254037844387076, 1.000000000000000000, 0.8660254037844387076, 1.000000000000000000, 0.8660254037844387076, 1.000000000000000000, 0.8660254037844387076, 1.000000000000000000, 0.8660254037844387076, 1.000000000000000000, 0.8660254037844387076, 1.000000000000000000, 0.8660254037844387076, 1.000000000000000000, 0.8660254037844387076, 1.000000000000000000, 0.8660254037844387076, 1.000000000000000000, 0.8660254037844387076, 1.000000000000000000, 0.8660254037844387076, 1.000000000000000000, 0.8660254037844387076, 1.000000000000000000, 0.8660254037844387076, 1.000000000000000000, 0.8660254037844387076, 1.000000000000000000, 0.8660254037844387076, 1.000000000000000000, 0.8660254037844387076, 1.000000000000000000, 0.8660254037844387076, 1.000000000000000000, 0.8660254037844387076, 1.000000000000000000, 0.8660254037844387076, 1.000000000000000000, 0.8660254037844387076, 1.000000000000000000, 0.8660254037844387076, 1.000000000000000000, 0.8660254037844387076, 1.000000000000000000, 0.8660254037844387076, 1.000000000000000000, 0.8660254037844387076, 1.000000000000000000, 0.8660254037844387076, 1.000000000000000000),
 ( 1.000000000000000000, 0.8660254037844387076, 1.000000000000000000, 0.8660254037844387076, 1.000000000000000000, 0.8660254037844387076, 1.000000000000000000, 0.8660254037844387076, 1.000000000000000000, 0.8660254037844387076, 1.000000000000000000, 0.8660254037844387076, 1.000000000000000000, 0.8660254037844387076, 1.000000000000000000, 0.8660254037844387076, 1.000000000000000000, 0.8660254037844387076, 1.000000000000000000, 0.8660254037844387076, 1.000000000000000000, 0.8660254037844387076, 1.000000000000000000, 0.8660254037844387076, 1.000000000000000000, 0.8660254037844387076, 1.000000000000000000, 0.8660254037844387076, 1.000000000000000000, 0.8660254037844387076, 1.000000000000000000, 0.8660254037844387076, 1.000000000000000000, 0.8660254037844387076, 1.000000000000000000, 0.8660254037844387076, 1.000000000000000000, 0.8660254037844387076, 1.000000000000000000, 0.8660254037844387076, 1.000000000000000000, 0.8660254037844387076, 1.000000000000000000, 0.8660254037844387076, 1.000000000000000000, 0.8660254037844387076, 1.000000000000000000, 0.8660254037844387076, 1.000000000000000000, 0.8660254037844387076, 1.000000000000000000, 0.8660254037844387076, 1.000000000000000000, 0.8660254037844387076, 1.000000000000000000, 0.8660254037844387076, 1.000000000000000000, 0.8660254037844387076, 1.000000000000000000, 0.8660254037844387076, 1.000000000000000000, 0.8660254037844387076, 1.000000000000000000, 0.8660254037844387076, 1.000000000000000000, 0.8660254037844387076, 1.000000000000000000, 0.8660254037844387076, 1.000000000000000000, 0.8660254037844387076, 1.000000000000000000, 0.8660254037844387076, 1.000000000000000000, 0.8660254037844387076, 1.000000000000000000, 0.8660254037844387076, 1.000000000000000000, 0.8660254037844387076, 1.000000000000000000, 0.8660254037844387076, 1.000000000000000000, 0.8660254037844387076, 1.000000000000000000, 0.8660254037844387076, 1.000000000000000000, 0.8660254037844387076, 1.000000000000000000, 0.8660254037844387076, 1.000000000000000000, 0.8660254037844387076, 1.000000000000000000, 0.8660254037844387076, 1.000000000000000000, 0.8660254037844387076, 1.000000000000000000, 0.8660254037844387076, 1.000000000000000000, 0.8660254037844387076, 1.000000000000000000, 0.8660254037844387076, 1.000000000000000000, 0.8660254037844387076, 1.000000000000000000, 0.8660254037844387076, 1.000000000000000000, 0.8660254037844387076, 1.000000000000000000, 0.8660254037844387076, 1.000000000000000000, 0.8660254037844387076, 1.000000000000000000, 0.8660254037844387076, 1.000000000000000000, 0.8660254037844387076, 1.000000000000000000, 0.8660254037844387076, 1.000000000000000000, 0.8660254037844387076, 1.000000000000000000, 0.8660254037844387076, 1.000000000000000000, 0.8660254037844387076, 1.000000000000000000, 0.8660254037844387076, 1.000000000000000000, 0.8660254037844387076, 1.000000000000000000, 0.8660254037844387076, 1.000000000000000000, 0.8660254037844387076, 1.000000000000000000, 0.8660254037844387076, 1.000000000000000000, 0.8660254037844387076, 1.000000000000000000, 0.8660254037844387076, 1.000000000000000000, 0.8660254037844387076, 1.000000000000000000, 0.8660254037844387076, 1.000000000000000000, 0.8660254037844387076, 1.000000000000000000, 0.8660254037844387076, 1.000000000000000000) ) ) 
 REPRESENTATION_ITEM ( '' )  SURFACE ( )  );
#819=CARTESIAN_POINT ( 'NONE',  ( 5.114683531250000748, -26.85937500034139802, 0.000000000000000000 ) ) ;
#826=ADVANCED_FACE ( 'NONE', ( #3906 ), #1011, .T. ) ;
#828=CARTESIAN_POINT ( 'NONE',  ( -1.406733260263385521, -27.82366454968462932, 5.250000000000006217 ) ) ;
#832=ORIENTED_EDGE ( 'NONE', *, *, #1444, .F. ) ;
#833=CARTESIAN_POINT ( 'NONE',  ( 0.000000000000000000, -30.00000000000000000, 0.000000000000000000 ) ) ;
#836=CARTESIAN_POINT ( 'NONE',  ( -5.250000000000000000, -29.39583333333332860, -3.031088913245536531 ) ) ;
#837=CARTESIAN_POINT ( 'NONE',  ( 3.616337804771879580E-16, -27.35937500034139802, -5.905927827173866440 ) ) ;
#838=CARTESIAN_POINT ( 'NONE',  ( -5.114683531250000748, -27.79687500034139802, -6.263680815196995234E-16 ) ) ;
#848=CARTESIAN_POINT ( 'NONE',  ( 5.114683531249999859, -28.83854166700806587, -2.952963913586932776 ) ) ;
#849=VERTEX_POINT ( 'NONE', #7295 ) ;
#853=CARTESIAN_POINT ( 'NONE',  ( 2.624999999999996891, -26.82291666734946389, 4.546633369868304797 ) ) ;
#858=CARTESIAN_POINT ( 'NONE',  ( -2.625000000000002220, -29.61458333401613174, 4.546633369868302132 ) ) ;
#861=CARTESIAN_POINT ( 'NONE',  ( 2.557341765625000818, -27.81770833367473017, -4.429445870380400052 ) ) ;
#870=VECTOR ( 'NONE', #6866, 1000.000000000000000 ) ;
#874=VERTEX_POINT ( 'NONE', #312 ) ;
#879=EDGE_LOOP ( 'NONE', ( #5757, #6091 ) ) ;
#881=CYLINDRICAL_SURFACE ( 'NONE', #3176, 5.250000000000000000 ) ;
#884=CARTESIAN_POINT ( 'NONE',  ( -5.250000000000000888, -29.10416666666666785, 3.031088913245532979 ) ) ;
#887=CARTESIAN_POINT ( 'NONE',  ( -1.084901341431563726E-15, -27.23437500034139802, 5.905927827173866440 ) ) ;
#888=AXIS2_PLACEMENT_3D ( 'NONE', #4026, #9081, #6861 ) ;
#891=CARTESIAN_POINT ( 'NONE',  ( -2.557341765624999042, -29.77604166700806232, -4.429445870380400052 ) ) ;
#895=DIRECTION ( 'NONE',  ( 0.000000000000000000, 1.000000000000000000, 0.000000000000000000 ) ) ;
#898=CARTESIAN_POINT ( 'NONE',  ( 1.406733260263402174, -27.08258545099816672, 5.249999999999995559 ) ) ;
#900=CARTESIAN_POINT ( 'NONE',  ( -5.114683531250000748, -28.23437500034139447, -6.263680815196995234E-16 ) ) ;
#902=ORIENTED_EDGE ( 'NONE', *, *, #6341, .F. ) ;
#905=EDGE_CURVE ( 'NONE', #8760, #6742, #5895, .T. ) ;
#907=CARTESIAN_POINT ( 'NONE',  ( 2.625000000000000444, -27.45833333333333215, -4.546633369868303021 ) ) ;
#908=ORIENTED_EDGE ( 'NONE', *, *, #7926, .T. ) ;
#912=CARTESIAN_POINT ( 'NONE',  ( -5.114683531250000748, -29.79687500034139802, -6.263680815196995234E-16 ) ) ;
#926=DIRECTION ( 'NONE',  ( 0.000000000000000000, 1.000000000000000000, 0.000000000000000000 ) ) ;
#930=AXIS2_PLACEMENT_3D ( 'NONE', #8253, #4020, #5403 ) ;
#932=CARTESIAN_POINT ( 'NONE',  ( -1.113604000661152470E-15, -27.81250000000000000, 6.062177826491070398 ) ) ;
#934=CARTESIAN_POINT ( 'NONE',  ( -5.114683531250001636, -28.52604166700806587, 2.952963913586931444 ) ) ;
#937=FILL_AREA_STYLE ('',( #5863 ) ) ;
#939=CARTESIAN_POINT ( 'NONE',  ( 0.000000000000000000, -30.00000000000000000, 0.000000000000000000 ) ) ;
#943=CARTESIAN_POINT ( 'NONE',  ( 5.114683531249999859, -28.40104166700806232, -2.952963913586932776 ) ) ;
#944=DIRECTION ( 'NONE',  ( 0.000000000000000000, 1.000000000000000000, 0.000000000000000000 ) ) ;
#947=CARTESIAN_POINT ( 'NONE',  ( 2.624999999999996891, -27.07291666734946389, 4.546633369868304797 ) ) ;
#948=CARTESIAN_POINT ( 'NONE',  ( -5.114683531250000748, -28.98437500034139802, -6.263680815196995234E-16 ) ) ;
#953=CARTESIAN_POINT ( 'NONE',  ( -1.406733260263387963, -29.17633545031536713, -5.250000000000001776 ) ) ;
#954=ORIENTED_EDGE ( 'NONE', *, *, #1054, .F. ) ;
#956=CARTESIAN_POINT ( 'NONE',  ( -2.625000000000002220, -28.86458333401612819, 4.546633369868302132 ) ) ;
#959=CARTESIAN_POINT ( 'NONE',  ( 5.114683531250000748, -27.35937500034139802, 0.000000000000000000 ) ) ;
#960=ORIENTED_EDGE ( 'NONE', *, *, #7717, .F. ) ;
#963=DIRECTION ( 'NONE',  ( 0.000000000000000000, 1.000000000000000000, 0.000000000000000000 ) ) ;
#977=VERTEX_POINT ( 'NONE', #4824 ) ;
#978=CARTESIAN_POINT ( 'NONE',  ( 3.712013335537174572E-16, -28.18749999999999645, -6.062177826491070398 ) ) ;
#980=CARTESIAN_POINT ( 'NONE',  ( -2.324088772396477476E-15, -29.46875000068279959, -5.250000000000000000 ) ) ;
#981=CARTESIAN_POINT ( 'NONE',  ( -2.557341765624999042, -28.52604166700806587, -4.429445870380400052 ) ) ;
#984=CARTESIAN_POINT ( 'NONE',  ( 5.249999999999997335, -28.80208333401612819, 3.031088913245538308 ) ) ;
#986=CARTESIAN_POINT ( 'NONE',  ( -5.114683531250000748, -29.04687500034139802, -6.263680815196995234E-16 ) ) ;
#988=ORIENTED_EDGE ( 'NONE', *, *, #517, .T. ) ;
#990=CARTESIAN_POINT ( 'NONE',  ( -5.114683531250000748, -28.46354166700806587, 2.952963913586931888 ) ) ;
#993=CYLINDRICAL_SURFACE ( 'NONE', #5848, 5.250000000000000000 ) ;
#1001=CARTESIAN_POINT ( 'NONE',  ( 0.000000000000000000, -30.00000000000000000, 0.000000000000000000 ) ) ;
#1004=CARTESIAN_POINT ( 'NONE',  ( -5.114683531249999859, -29.06770833367473017, -2.952963913586935440 ) ) ;
#1006=DIRECTION ( 'NONE',  ( 0.000000000000000000, 1.000000000000000000, 0.000000000000000000 ) ) ;
#1008=DIRECTION ( 'NONE',  ( 0.000000000000000000, 0.000000000000000000, 1.000000000000000000 ) ) ;
#1011=CYLINDRICAL_SURFACE ( 'NONE', #6584, 5.250000000000000000 ) ;
#1014=CYLINDRICAL_SURFACE ( 'NONE', #6247, 5.750000000000000000 ) ;
#1023=CARTESIAN_POINT ( 'NONE',  ( 2.624999999999996891, -28.04166666666666785, 4.546633369868304797 ) ) ;
#1024=AXIS2_PLACEMENT_3D ( 'NONE', #6724, #963, #8824 ) ;
#1030=CARTESIAN_POINT ( 'NONE',  ( 5.114683531249998971, -28.38020833367473017, 2.952963913586936329 ) ) ;
#1033=CARTESIAN_POINT ( 'NONE',  ( -1.975475456537005874E-15, -27.56249999999999289, 5.249999999999999112 ) ) ;
#1034=CARTESIAN_POINT ( 'NONE',  ( -2.557341765625002594, -28.50520833367473017, 4.429445870380399164 ) ) ;
#1037=CARTESIAN_POINT ( 'NONE',  ( 5.114683531249998971, -27.63020833367473017, 2.952963913586936329 ) ) ;
#1039=( BOUNDED_CURVE ( )  B_SPLINE_CURVE ( 2, ( #3080, #1723, #3126, #5902, #2469, #8789, #8741, #5856, #8144 ),
 .UNSPECIFIED., .F., .F. ) 
 B_SPLINE_CURVE_WITH_KNOTS ( ( 3, 2, 2, 2, 3 ),
 ( 0.8541666666666666297, 0.8611111111111111605, 0.8750000000000000000, 0.8888888888888888395, 0.8958333333333333703 ),
 .UNSPECIFIED. ) 
 CURVE ( )  GEOMETRIC_REPRESENTATION_ITEM ( )  RATIONAL_B_SPLINE_CURVE ( ( 0.9330127018922192983, 0.9330127018922187432, 1.000000000000000000, 0.8660254037844387076, 1.000000000000000000, 0.8660254037844387076, 1.000000000000000000, 0.9330127018922187432, 0.9330127018922192983 ) ) 
 REPRESENTATION_ITEM ( '' )  );
#1043=ADVANCED_FACE ( 'NONE', ( #1954 ), #6130, .T. ) ;
#1046=DIRECTION ( 'NONE',  ( 0.000000000000000000, 1.000000000000000000, 0.000000000000000000 ) ) ;
#1049=VECTOR ( 'NONE', #483, 1000.000000000000000 ) ;
#1050=EDGE_CURVE ( 'NONE', #7374, #3248, #5428, .T. ) ;
#1051=CARTESIAN_POINT ( 'NONE',  ( 1.406733260263391960, -29.33258545099816317, 5.250000000000000000 ) ) ;
#1052=CARTESIAN_POINT ( 'NONE',  ( 5.250000000000000000, -28.01041666734946389, -3.031088913245534755 ) ) ;
#1054=EDGE_CURVE ( 'NONE', #2054, #7800, #8781, .T. ) ;
#1056=VERTEX_POINT ( 'NONE', #3998 ) ;
#1060=CYLINDRICAL_SURFACE ( 'NONE', #433, 2.750000000000000000 ) ;
#1062=CARTESIAN_POINT ( 'NONE',  ( 5.114683531250000748, -29.92187500034139802, 0.000000000000000000 ) ) ;
#1064=CARTESIAN_POINT ( 'NONE',  ( 3.616337804771879580E-16, -29.54687500034139802, -5.905927827173866440 ) ) ;
#1075=CARTESIAN_POINT ( 'NONE',  ( -5.250000000000000888, -27.35416666666666430, 3.031088913245532979 ) ) ;
#1076=CARTESIAN_POINT ( 'NONE',  ( -5.250000000000000888, -28.63541666734946389, 3.031088913245533423 ) ) ;
#1078=CARTESIAN_POINT ( 'NONE',  ( -1.084901341431563726E-15, -26.98437500034139802, 5.905927827173866440 ) ) ;
#1080=( LENGTH_UNIT ( ) NAMED_UNIT ( * ) SI_UNIT ( .MILLI., .METRE. ) );
#1083=CARTESIAN_POINT ( 'NONE',  ( 2.557341765625000818, -28.81770833367473017, -4.429445870380400052 ) ) ;
#1087=CARTESIAN_POINT ( 'NONE',  ( -2.557341765624999042, -29.08854166700806587, -4.429445870380400052 ) ) ;
#1089=AXIS2_PLACEMENT_3D ( 'NONE', #939, #8612, #148 ) ;
#1091=CARTESIAN_POINT ( 'NONE',  ( -2.557341765624999042, -27.27604166700806587, -4.429445870380400052 ) ) ;
#1103=CARTESIAN_POINT ( 'NONE',  ( -2.624999999999998668, -27.44791666734946389, -4.546633369868303021 ) ) ;
#1109=CARTESIAN_POINT ( 'NONE',  ( -1.975475456537005874E-15, -29.06249999999999645, 5.249999999999999112 ) ) ;
#1110=ADVANCED_FACE ( 'NONE', ( #1205 ), #4091, .F. ) ;
#1112=DIRECTION ( 'NONE',  ( 0.000000000000000000, 1.000000000000000000, 0.000000000000000000 ) ) ;
#1114=CARTESIAN_POINT ( 'NONE',  ( -5.114683531250000748, -29.46354166700806232, 2.952963913586931888 ) ) ;
#1122=EDGE_LOOP ( 'NONE', ( #3146, #1512, #5729, #3838 ) ) ;
#1123=CARTESIAN_POINT ( 'NONE',  ( 2.624999999999996891, -27.79166666666666430, 4.546633369868304797 ) ) ;
#1127=( BOUNDED_CURVE ( )  B_SPLINE_CURVE ( 2, ( #482, #6057, #431, #8207, #385, #4579, #7725, #8893, #2536 ),
 .UNSPECIFIED., .F., .T. ) 
 B_SPLINE_CURVE_WITH_KNOTS ( ( 3, 2, 2, 2, 3 ),
 ( 0.6041666666666666297, 0.6111111111111111605, 0.6250000000000000000, 0.6388888888888888395, 0.6458333333333333703 ),
 .UNSPECIFIED. ) 
 CURVE ( )  GEOMETRIC_REPRESENTATION_ITEM ( )  RATIONAL_B_SPLINE_CURVE ( ( 0.9330127018922192983, 0.9330127018922187432, 1.000000000000000000, 0.8660254037844387076, 1.000000000000000000, 0.8660254037844387076, 1.000000000000000000, 0.9330127018922187432, 0.9330127018922192983 ) ) 
 REPRESENTATION_ITEM ( '' )  );
#1131=CARTESIAN_POINT ( 'NONE',  ( 5.114683531249998971, -28.63020833367473017, 2.952963913586936329 ) ) ;
#1133=CARTESIAN_POINT ( 'NONE',  ( 1.406733260263397289, -28.58258545099816672, 5.249999999999997335 ) ) ;
#1135=CARTESIAN_POINT ( 'NONE',  ( 2.557341765624996821, -28.46354166700806587, 4.429445870380401828 ) ) ;
#1138=CARTESIAN_POINT ( 'NONE',  ( 2.557341765625000818, -27.31770833367473017, -4.429445870380400052 ) ) ;
#1142=CARTESIAN_POINT ( 'NONE',  ( -1.406733260263390628, -28.57366454968462577, 5.250000000000001776 ) ) ;
#1148=CARTESIAN_POINT ( 'NONE',  ( -1.113604000661152470E-15, -28.09375000068279249, 6.062177826491070398 ) ) ;
#1154=CARTESIAN_POINT ( 'NONE',  ( 2.300847884672513123E-14, -28.18750000000000000, -5.250000000000000000 ) ) ;
#1156=CARTESIAN_POINT ( 'NONE',  ( 1.406733260263393070, -29.69866454968462577, -5.250000000000000888 ) ) ;
#1157=ORIENTED_EDGE ( 'NONE', *, *, #4558, .T. ) ;
#1165=EDGE_CURVE ( 'NONE', #1550, #8808, #7578, .T. ) ;
#1175=CARTESIAN_POINT ( 'NONE',  ( 3.616337804771879580E-16, -29.29687500034139802, -5.905927827173866440 ) ) ;
#1177=CARTESIAN_POINT ( 'NONE',  ( 0.000000000000000000, -30.00000000000000000, 0.000000000000000000 ) ) ;
#1178=CARTESIAN_POINT ( 'NONE',  ( -2.557341765625002594, -27.00520833367473017, 4.429445870380399164 ) ) ;
#1179=( BOUNDED_CURVE ( )  B_SPLINE_CURVE ( 2, ( #782, #5710, #8553, #2979, #7859, #5002, #1480, #4324, #7203 ),
 .UNSPECIFIED., .F., .F. ) 
 B_SPLINE_CURVE_WITH_KNOTS ( ( 3, 2, 2, 2, 3 ),
 ( 0.6875000000000000000, 0.6944444444444444198, 0.7083333333333333703, 0.7222222222222222099, 0.7291666666666667407 ),
 .UNSPECIFIED. ) 
 CURVE ( )  GEOMETRIC_REPRESENTATION_ITEM ( )  RATIONAL_B_SPLINE_CURVE ( ( 0.9330127018922194093, 0.9330127018922194093, 1.000000000000000000, 0.8660254037844387076, 1.000000000000000000, 0.8660254037844387076, 1.000000000000000000, 0.9330127018922187432, 0.9330127018922192983 ) ) 
 REPRESENTATION_ITEM ( '' )  );
#1181=CARTESIAN_POINT ( 'NONE',  ( -1.084901341431563923E-15, -27.17187500034140157, 5.905927827173866440 ) ) ;
#1183=CARTESIAN_POINT ( 'NONE',  ( 5.114683531250000748, -28.67187500034139802, 0.000000000000000000 ) ) ;
#1187=FACE_BOUND ( 'NONE', #3193, .T. ) ;
#1188=FACE_OUTER_BOUND ( 'NONE', #7727, .T. ) ;
#1193=ORIENTED_EDGE ( 'NONE', *, *, #1508, .F. ) ;
#1195=CARTESIAN_POINT ( 'NONE',  ( 2.624999999999996891, -29.32291666734946034, 4.546633369868304797 ) ) ;
#1196=CARTESIAN_POINT ( 'NONE',  ( -5.250000000000000000, -28.65625000068279604, -6.429395695523604153E-16 ) ) ;
#1200=VERTEX_POINT ( 'NONE', #7011 ) ;
#1205=FACE_OUTER_BOUND ( 'NONE', #2938, .T. ) ;
#1211=CARTESIAN_POINT ( 'NONE',  ( 5.182341765625000818, -29.82031250051209881, 0.000000000000000000 ) ) ;
#1217=CARTESIAN_POINT ( 'NONE',  ( 2.624999999999996891, -27.04166666666666430, 4.546633369868304797 ) ) ;
#1223=CARTESIAN_POINT ( 'NONE',  ( 2.557341765624996821, -28.15104166700806587, 4.429445870380401828 ) ) ;
#1225=CARTESIAN_POINT ( 'NONE',  ( 0.000000000000000000, -30.00000000000000000, 0.000000000000000000 ) ) ;
#1226=CARTESIAN_POINT ( 'NONE',  ( -2.557341765624999042, -27.58854166700806587, -4.429445870380400052 ) ) ;
#1227=DIRECTION ( 'NONE',  ( 0.000000000000000000, 0.000000000000000000, 1.000000000000000000 ) ) ;
#1229=CARTESIAN_POINT ( 'NONE',  ( -5.114683531250000748, -27.71354166700806587, 2.952963913586931888 ) ) ;
#1231=CARTESIAN_POINT ( 'NONE',  ( 2.557341765625000818, -29.38020833367473017, -4.429445870380400052 ) ) ;
#1239=AXIS2_PLACEMENT_3D ( 'NONE', #1225, #6705, #6155 ) ;
#1240=ORIENTED_EDGE ( 'NONE', *, *, #8391, .F. ) ;
#1242=CARTESIAN_POINT ( 'NONE',  ( 5.250000000000000000, -28.51041666734946389, -3.031088913245534755 ) ) ;
#1244=CIRCLE ( 'NONE', #500, 2.750000000000000000 ) ;
#1250=CARTESIAN_POINT ( 'NONE',  ( 5.249999999999999112, -29.47916666666666430, -3.031088913245534755 ) ) ;
#1255=CARTESIAN_POINT ( 'NONE',  ( -2.324088772396477476E-15, -29.68750000000000000, -5.250000000000000000 ) ) ;
#1256=DIRECTION ( 'NONE',  ( 0.000000000000000000, 0.000000000000000000, 1.000000000000000000 ) ) ;
#1269=CARTESIAN_POINT ( 'NONE',  ( -5.114683531250001636, -27.46354166700806587, 2.952963913586931444 ) ) ;
#1272=CARTESIAN_POINT ( 'NONE',  ( 3.712013335537174572E-16, -29.93749999999999645, -6.062177826491070398 ) ) ;
#1274=CARTESIAN_POINT ( 'NONE',  ( -2.557341765625002594, -29.00520833367473017, 4.429445870380399164 ) ) ;
#1275=CARTESIAN_POINT ( 'NONE',  ( -2.557341765625002594, -29.50520833367473017, 4.429445870380399164 ) ) ;
#1284=CARTESIAN_POINT ( 'NONE',  ( 5.250000000000000000, -27.26041666734946034, -3.031088913245534755 ) ) ;
#1289=DIRECTION ( 'NONE',  ( 0.000000000000000000, 0.000000000000000000, 1.000000000000000000 ) ) ;
#1292=CARTESIAN_POINT ( 'NONE',  ( -1.975475456537005874E-15, -28.31249999999999645, 5.250000000000000000 ) ) ;
#1294=CARTESIAN_POINT ( 'NONE',  ( -5.114683531250000748, -28.96354166700807298, 2.952963913586931888 ) ) ;
#1298=DIRECTION ( 'NONE',  ( 0.000000000000000000, 0.000000000000000000, 1.000000000000000000 ) ) ;
#1299=COLOUR_RGB ( '',0.8941176470588234615, 0.8941176470588234615, 0.8941176470588234615 ) ;
#1302=CARTESIAN_POINT ( 'NONE',  ( -5.250000000000000888, -27.10416666666666430, 3.031088913245532979 ) ) ;
#1308=CARTESIAN_POINT ( 'NONE',  ( -5.114683531250000748, -27.50520833367473017, -2.952963913586935440 ) ) ;
#1310=CARTESIAN_POINT ( 'NONE',  ( -5.114683531250000748, -27.52604166700806587, 2.952963913586931888 ) ) ;
#1311=CARTESIAN_POINT ( 'NONE',  ( 6.972266317189433020E-16, -27.93749999999999289, -5.250000000000000000 ) ) ;
#1313=CARTESIAN_POINT ( 'NONE',  ( 5.114683531249998971, -28.94270833367473017, 2.952963913586936329 ) ) ;
#1316=CARTESIAN_POINT ( 'NONE',  ( -1.084901341431563923E-15, -28.48437500034139802, 5.905927827173866440 ) ) ;
#1317=CARTESIAN_POINT ( 'NONE',  ( 6.429395695523604153E-16, -30.00000000000000000, -5.250000000000000000 ) ) ;
#1320=CARTESIAN_POINT ( 'NONE',  ( -2.324088772396477476E-15, -29.46875000068279959, -5.250000000000000000 ) ) ;
#1324=ORIENTED_EDGE ( 'NONE', *, *, #8892, .T. ) ;
#1325=VECTOR ( 'NONE', #2363, 1000.000000000000000 ) ;
#1327=CARTESIAN_POINT ( 'NONE',  ( 2.557341765625000818, -29.31770833367473017, -4.429445870380400052 ) ) ;
#1341=CARTESIAN_POINT ( 'NONE',  ( -5.114683531250000748, -27.96354166700806587, 2.952963913586931888 ) ) ;
#1344=CARTESIAN_POINT ( 'NONE',  ( 5.249999999999997335, -29.05208333401613174, 3.031088913245538308 ) ) ;
#1346=( BOUNDED_CURVE ( )  B_SPLINE_CURVE ( 2, ( #6435, #2875, #1377, #3478, #5606, #5565, #3520, #6305, #9097 ),
 .UNSPECIFIED., .F., .F. ) 
 B_SPLINE_CURVE_WITH_KNOTS ( ( 3, 2, 2, 2, 3 ),
 ( 0.9375000000000000000, 0.9444444444444444198, 0.9583333333333333703, 0.9722222222222222099, 0.9791666666666667407 ),
 .UNSPECIFIED. ) 
 CURVE ( )  GEOMETRIC_REPRESENTATION_ITEM ( )  RATIONAL_B_SPLINE_CURVE ( ( 0.9330127018922194093, 0.9330127018922194093, 1.000000000000000000, 0.8660254037844387076, 1.000000000000000000, 0.8660254037844387076, 1.000000000000000000, 0.9330127018922187432, 0.9330127018922192983 ) ) 
 REPRESENTATION_ITEM ( '' )  );
#1350=CARTESIAN_POINT ( 'NONE',  ( 1.185285273922203525E-14, -28.93749999999999645, -5.250000000000000000 ) ) ;
#1356=CARTESIAN_POINT ( 'NONE',  ( -1.084901341431563726E-15, -27.67187500034140157, 5.905927827173866440 ) ) ;
#1358=CARTESIAN_POINT ( 'NONE',  ( 5.114683531249998971, -27.19270833367473017, 2.952963913586936329 ) ) ;
#1359=DIRECTION ( 'NONE',  ( 0.000000000000000000, 1.000000000000000000, 0.000000000000000000 ) ) ;
#1361=CARTESIAN_POINT ( 'NONE',  ( -1.084901341431563726E-15, -29.73437500034140513, 5.905927827173866440 ) ) ;
#1363=CARTESIAN_POINT ( 'NONE',  ( 5.114683531250000748, -27.92187500034139802, 0.000000000000000000 ) ) ;
#1364=CARTESIAN_POINT ( 'NONE',  ( -5.250000000000000000, -29.62500000000000000, -6.429395695523604153E-16 ) ) ;
#1371=EDGE_LOOP ( 'NONE', ( #5607, #6567, #6671, #3159 ) ) ;
#1373=CARTESIAN_POINT ( 'NONE',  ( -5.114683531249999859, -29.25520833367473017, -2.952963913586935440 ) ) ;
#1374=VERTEX_POINT ( 'NONE', #9144 ) ;
#1377=CARTESIAN_POINT ( 'NONE',  ( -2.624999999999998668, -27.16666666666666430, -4.546633369868303021 ) ) ;
#1378=VERTEX_POINT ( 'NONE', #8543 ) ;
#1382=CARTESIAN_POINT ( 'NONE',  ( 5.114683531250000748, -28.35937500034139447, 0.000000000000000000 ) ) ;
#1383=CARTESIAN_POINT ( 'NONE',  ( 6.429395695523604153E-16, -30.00000000000000000, -5.250000000000000000 ) ) ;
#1388=AXIS2_PLACEMENT_3D ( 'NONE', #217, #4363, #5844 ) ;
#1391=AXIS2_PLACEMENT_3D ( 'NONE', #2767, #1359, #9161 ) ;
#1393=LINE ( 'NONE', #9153, #2840 ) ;
#1394=( BOUNDED_CURVE ( )  B_SPLINE_CURVE ( 2, ( #4872, #2888, #8549, #6490, #2046, #5750, #3489, #2797, #6356 ),
 .UNSPECIFIED., .F., .F. ) 
 B_SPLINE_CURVE_WITH_KNOTS ( ( 3, 2, 2, 2, 3 ),
 ( 0.5208333333333332593, 0.5277777777777777901, 0.5416666666666666297, 0.5555555555555555802, 0.5625000000000000000 ),
 .UNSPECIFIED. ) 
 CURVE ( )  GEOMETRIC_REPRESENTATION_ITEM ( )  RATIONAL_B_SPLINE_CURVE ( ( 0.9330127018922192983, 0.9330127018922187432, 1.000000000000000000, 0.8660254037844387076, 1.000000000000000000, 0.8660254037844387076, 1.000000000000000000, 0.9330127018922194093, 0.9330127018922194093 ) ) 
 REPRESENTATION_ITEM ( '' )  );
#1395=ORIENTED_EDGE ( 'NONE', *, *, #4836, .T. ) ;
#1399=CARTESIAN_POINT ( 'NONE',  ( -5.114683531250000748, -27.23437500034139802, -6.263680815196995234E-16 ) ) ;
#1401=CARTESIAN_POINT ( 'NONE',  ( 3.712013335537174572E-16, -28.68749999999999645, -6.062177826491070398 ) ) ;
#1404=CARTESIAN_POINT ( 'NONE',  ( -2.557341765624999042, -29.08854166700806587, -4.429445870380400052 ) ) ;
#1406=CARTESIAN_POINT ( 'NONE',  ( 3.616337804771879580E-16, -27.10937500034139802, -5.905927827173866440 ) ) ;
#1412=CARTESIAN_POINT ( 'NONE',  ( 6.972266317189433020E-16, -29.71875000068279249, -5.250000000000000000 ) ) ;
#1415=CARTESIAN_POINT ( 'NONE',  ( 3.616337804771879580E-16, -29.54687500034139802, -5.905927827173866440 ) ) ;
#1416=( BOUNDED_CURVE ( )  B_SPLINE_CURVE ( 2, ( #1311, #1432, #7906, #5667, #2141, #5805, #4415, #828, #44 ),
 .UNSPECIFIED., .F., .T. ) 
 B_SPLINE_CURVE_WITH_KNOTS ( ( 3, 2, 2, 2, 3 ),
 ( 0.6875000000000000000, 0.6944444444444444198, 0.7083333333333333703, 0.7222222222222222099, 0.7291666666666667407 ),
 .UNSPECIFIED. ) 
 CURVE ( )  GEOMETRIC_REPRESENTATION_ITEM ( )  RATIONAL_B_SPLINE_CURVE ( ( 0.9330127018922194093, 0.9330127018922194093, 1.000000000000000000, 0.8660254037844387076, 1.000000000000000000, 0.8660254037844387076, 1.000000000000000000, 0.9330127018922187432, 0.9330127018922192983 ) ) 
 REPRESENTATION_ITEM ( '' )  );
#1421=ORIENTED_EDGE ( 'NONE', *, *, #9098, .F. ) ;
#1424=CARTESIAN_POINT ( 'NONE',  ( 2.624999999999996891, -27.82291666734946389, 4.546633369868304797 ) ) ;
#1425=CARTESIAN_POINT ( 'NONE',  ( 5.114683531249998971, -28.38020833367473372, 2.952963913586936329 ) ) ;
#1426=CARTESIAN_POINT ( 'NONE',  ( 2.625000000000000444, -27.48958333401612819, -4.546633369868303021 ) ) ;
#1427=CARTESIAN_POINT ( 'NONE',  ( -2.624999999999998668, -28.94791666734946389, -4.546633369868303021 ) ) ;
#1432=CARTESIAN_POINT ( 'NONE',  ( -1.406733260263393293, -27.92633545031536713, -5.250000000000000000 ) ) ;
#1437=CARTESIAN_POINT ( 'NONE',  ( -5.114683531250000748, -26.98437500034139802, -6.263680815196995234E-16 ) ) ;
#1439=VERTEX_POINT ( 'NONE', #3570 ) ;
#1440=CARTESIAN_POINT ( 'NONE',  ( 5.249999999999999112, -29.02083333333333570, 3.031088913245538308 ) ) ;
#1443=CARTESIAN_POINT ( 'NONE',  ( -5.114683531250001636, -29.52604166700806232, 2.952963913586931444 ) ) ;
#1444=EDGE_CURVE ( 'NONE', #7933, #3802, #2311, .T. ) ;
#1445=CARTESIAN_POINT ( 'NONE',  ( -5.114683531249999859, -27.81770833367473017, -2.952963913586935440 ) ) ;
#1450=FACE_OUTER_BOUND ( 'NONE', #5236, .T. ) ;
#1451=CARTESIAN_POINT ( 'NONE',  ( 0.000000000000000000, -30.00000000000000000, 0.000000000000000000 ) ) ;
#1453=EDGE_LOOP ( 'NONE', ( #2480, #5936, #1395, #6149 ) ) ;
#1456=CARTESIAN_POINT ( 'NONE',  ( 5.249999999999999112, -26.80208333401613174, 3.031088913245538308 ) ) ;
#1457=EDGE_LOOP ( 'NONE', ( #8075, #3517, #4280, #8793 ) ) ;
#1461=FACE_OUTER_BOUND ( 'NONE', #6409, .T. ) ;
#1468=ADVANCED_FACE ( 'NONE', ( #3803 ), #817, .T. ) ;
#1471=CARTESIAN_POINT ( 'NONE',  ( -5.114683531249999859, -29.00520833367473017, -2.952963913586935440 ) ) ;
#1475=DIRECTION ( 'NONE',  ( 0.000000000000000000, 1.000000000000000000, 0.000000000000000000 ) ) ;
#1480=CARTESIAN_POINT ( 'NONE',  ( -2.625000000000002220, -27.61458333401612819, 4.546633369868302132 ) ) ;
#1489=CARTESIAN_POINT ( 'NONE',  ( 5.250000000000000000, -28.74999999999999645, 0.000000000000000000 ) ) ;
#1491=CARTESIAN_POINT ( 'NONE',  ( 2.557341765624996821, -27.96354166700806587, 4.429445870380401828 ) ) ;
#1493=CARTESIAN_POINT ( 'NONE',  ( -2.557341765625002594, -27.75520833367473017, 4.429445870380399164 ) ) ;
#1494=CARTESIAN_POINT ( 'NONE',  ( -5.114683531250001636, -29.71354166700806232, 2.952963913586931444 ) ) ;
#1495=DIRECTION ( 'NONE',  ( 0.000000000000000000, 1.000000000000000000, 0.000000000000000000 ) ) ;
#1499=CARTESIAN_POINT ( 'NONE',  ( -5.250000000000000888, -29.63541666734946389, 3.031088913245533423 ) ) ;
#1502=CARTESIAN_POINT ( 'NONE',  ( -2.624999999999998668, -28.69791666734946389, -4.546633369868303021 ) ) ;
#1503=CARTESIAN_POINT ( 'NONE',  ( -5.250000000000000888, -29.35416666666666430, 3.031088913245533423 ) ) ;
#1504=CARTESIAN_POINT ( 'NONE',  ( 5.114683531249998971, -28.88020833367473017, 2.952963913586936329 ) ) ;
#1507=CARTESIAN_POINT ( 'NONE',  ( 0.000000000000000000, -30.00000000000000000, 0.000000000000000000 ) ) ;
#1508=EDGE_CURVE ( 'NONE', #3111, #3057, #6807, .T. ) ;
#1511=CARTESIAN_POINT ( 'NONE',  ( 6.972266317189433020E-16, -26.96875000068279249, -5.249999999999999112 ) ) ;
#1512=ORIENTED_EDGE ( 'NONE', *, *, #6392, .T. ) ;
#1513=CARTESIAN_POINT ( 'NONE',  ( -2.624999999999998668, -27.66666666666666430, -4.546633369868303021 ) ) ;
#1517=CARTESIAN_POINT ( 'NONE',  ( 5.114683531249999859, -27.33854166700806232, -2.952963913586932776 ) ) ;
#1521=CYLINDRICAL_SURFACE ( 'NONE', #2813, 5.750000000000000000 ) ;
#1525=CARTESIAN_POINT ( 'NONE',  ( 0.000000000000000000, -9.000000000000001776, 0.000000000000000000 ) ) ;
#1526=LINE ( 'NONE', #2181, #6846 ) ;
#1532=ORIENTED_EDGE ( 'NONE', *, *, #3503, .F. ) ;
#1535=ORIENTED_EDGE ( 'NONE', *, *, #517, .F. ) ;
#1536=CARTESIAN_POINT ( 'NONE',  ( -5.250000000000000000, -29.37500000000000000, -6.429395695523604153E-16 ) ) ;
#1538=EDGE_CURVE ( 'NONE', #813, #6454, #6058, .T. ) ;
#1540=CARTESIAN_POINT ( 'NONE',  ( -5.114683531250001636, -27.77604166700806587, 2.952963913586931444 ) ) ;
#1542=CARTESIAN_POINT ( 'NONE',  ( 3.616337804771879580E-16, -28.10937500034140157, -5.905927827173866440 ) ) ;
#1547=CARTESIAN_POINT ( 'NONE',  ( -1.975475456537005874E-15, -27.34375000068279249, 5.250000000000000000 ) ) ;
#1550=VERTEX_POINT ( 'NONE', #4069 ) ;
#1552=CARTESIAN_POINT ( 'NONE',  ( 5.249999999999999112, -27.97916666666666430, -3.031088913245534755 ) ) ;
#1553=CARTESIAN_POINT ( 'NONE',  ( 2.557341765625000818, -28.81770833367473017, -4.429445870380400052 ) ) ;
#1561=DIRECTION ( 'NONE',  ( 0.000000000000000000, 1.000000000000000000, 0.000000000000000000 ) ) ;
#1562=CARTESIAN_POINT ( 'NONE',  ( 2.624999999999996891, -29.32291666734946034, 4.546633369868304797 ) ) ;
#1564=CARTESIAN_POINT ( 'NONE',  ( 5.114683531249998971, -26.88020833367473017, 2.952963913586936329 ) ) ;
#1566=DIRECTION ( 'NONE',  ( 0.000000000000000000, 0.000000000000000000, 1.000000000000000000 ) ) ;
#1567=ADVANCED_FACE ( 'NONE', ( #8163 ), #7509, .T. ) ;
#1569=DIRECTION ( 'NONE',  ( 0.8660254037844402619, 0.4999999999999970579, -0.000000000000000000 ) ) ;
#1573=CARTESIAN_POINT ( 'NONE',  ( -2.624999999999998668, -26.94791666734946389, -4.546633369868303021 ) ) ;
#1575=EDGE_CURVE ( 'NONE', #803, #8842, #8724, .T. ) ;
#1581=CARTESIAN_POINT ( 'NONE',  ( -5.114683531250001636, -26.96354166700806232, 2.952963913586931444 ) ) ;
#1584=CARTESIAN_POINT ( 'NONE',  ( -5.250000000000000000, -28.87499999999999645, -6.429395695523604153E-16 ) ) ;
#1585=CARTESIAN_POINT ( 'NONE',  ( -5.114683531250001636, -28.27604166700806587, 2.952963913586931444 ) ) ;
#1588=CARTESIAN_POINT ( 'NONE',  ( 5.114683531250000748, -29.85937500034139802, 0.000000000000000000 ) ) ;
#1596=CARTESIAN_POINT ( 'NONE',  ( -1.406733260263393293, -29.42633545031537423, -5.250000000000000000 ) ) ;
#1597=CARTESIAN_POINT ( 'NONE',  ( -2.557341765625002594, -28.94270833367473017, 4.429445870380399164 ) ) ;
#1602=CARTESIAN_POINT ( 'NONE',  ( 5.250000000000000000, -27.50000000000000000, 0.000000000000000000 ) ) ;
#1605=CARTESIAN_POINT ( 'NONE',  ( -1.975475456537005874E-15, -29.81249999999999645, 5.250000000000000000 ) ) ;
#1606=DIRECTION ( 'NONE',  ( 0.000000000000000000, 1.000000000000000000, 0.000000000000000000 ) ) ;
#1609=CARTESIAN_POINT ( 'NONE',  ( -5.114683531249999859, -29.81770833367473017, -2.952963913586935440 ) ) ;
#1610=CARTESIAN_POINT ( 'NONE',  ( 1.406733260263405061, -27.47991455036742181, -5.249999999999994671 ) ) ;
#1611=VECTOR ( 'NONE', #1569, 1000.000000000000114 ) ;
#1615=FACE_OUTER_BOUND ( 'NONE', #3876, .T. ) ;
#1628=AXIS2_PLACEMENT_3D ( 'NONE', #5867, #799, #3688 ) ;
#1629=CARTESIAN_POINT ( 'NONE',  ( 5.114683531249998971, -26.88020833367473017, 2.952963913586936329 ) ) ;
#1632=CARTESIAN_POINT ( 'NONE',  ( -5.250000000000000000, -28.14583333333333215, -3.031088913245536531 ) ) ;
#1634=CARTESIAN_POINT ( 'NONE',  ( 3.616337804771879580E-16, -28.10937500034139802, -5.905927827173866440 ) ) ;
#1642=CARTESIAN_POINT ( 'NONE',  ( 5.249999999999997335, -28.77083333333333215, 3.031088913245538308 ) ) ;
#1643=CARTESIAN_POINT ( 'NONE',  ( 5.114683531249998971, -28.44270833367473017, 2.952963913586936329 ) ) ;
#1647=CARTESIAN_POINT ( 'NONE',  ( -5.249999999999999112, -28.67708333401612464, -3.031088913245536975 ) ) ;
#1648=CARTESIAN_POINT ( 'NONE',  ( 5.249999999999997335, -27.05208333401612819, 3.031088913245538308 ) ) ;
#1649=AXIS2_PLACEMENT_3D ( 'NONE', #4104, #3450, #8927 ) ;
#1650=CARTESIAN_POINT ( 'NONE',  ( 5.114683531249998971, -28.63020833367472662, 2.952963913586936329 ) ) ;
#1655=CARTESIAN_POINT ( 'NONE',  ( 1.406733260263391960, -27.55133545031536713, 5.250000000000000000 ) ) ;
#1656=EDGE_LOOP ( 'NONE', ( #1731, #692, #8798, #2540 ) ) ;
#1658=CARTESIAN_POINT ( 'NONE',  ( -1.113604000661152470E-15, -28.84375000068279959, 6.062177826491070398 ) ) ;
#1661=CARTESIAN_POINT ( 'NONE',  ( -1.084901341431563923E-15, -27.67187500034140157, 5.905927827173866440 ) ) ;
#1662=ORIENTED_EDGE ( 'NONE', *, *, #4479, .F. ) ;
#1675=ORIENTED_EDGE ( 'NONE', *, *, #4460, .T. ) ;
#1680=CARTESIAN_POINT ( 'NONE',  ( 3.712013335537174572E-16, -27.68750000000000000, -6.062177826491070398 ) ) ;
#1681=CARTESIAN_POINT ( 'NONE',  ( -2.557341765624999042, -28.33854166700806587, -4.429445870380400052 ) ) ;
#1684=( NAMED_UNIT ( * ) PLANE_ANGLE_UNIT ( ) SI_UNIT ( $, .RADIAN. ) );
#1690=CARTESIAN_POINT ( 'NONE',  ( 2.624999999999996891, -28.79166666666666785, 4.546633369868304797 ) ) ;
#1691=CARTESIAN_POINT ( 'NONE',  ( -2.557341765625002594, -29.25520833367473017, 4.429445870380399164 ) ) ;
#1692=CARTESIAN_POINT ( 'NONE',  ( 5.249999999999999112, -28.26041666734946745, -3.031088913245534755 ) ) ;
#1694=ORIENTED_EDGE ( 'NONE', *, *, #6925, .F. ) ;
#1696=CARTESIAN_POINT ( 'NONE',  ( 5.114683531249999859, -28.08854166700806232, -2.952963913586932776 ) ) ;
#1698=ORIENTED_EDGE ( 'NONE', *, *, #8246, .F. ) ;
#1699=CYLINDRICAL_SURFACE ( 'NONE', #1849, 5.250000000000000000 ) ;
#1702=CARTESIAN_POINT ( 'NONE',  ( -2.624999999999998668, -29.16666666666666785, -4.546633369868303021 ) ) ;
#1706=CARTESIAN_POINT ( 'NONE',  ( 2.625000000000000444, -28.73958333401612819, -4.546633369868303021 ) ) ;
#1708=CARTESIAN_POINT ( 'NONE',  ( -2.557341765624999042, -27.77604166700806587, -4.429445870380400052 ) ) ;
#1709=ORIENTED_EDGE ( 'NONE', *, *, #5661, .T. ) ;
#1710=FACE_OUTER_BOUND ( 'NONE', #3361, .T. ) ;
#1720=( BOUNDED_CURVE ( )  B_SPLINE_CURVE ( 2, ( #8620, #898, #947, #1648, #3748, #8576, #7222, #8668, #3835 ),
 .UNSPECIFIED., .F., .T. ) 
 B_SPLINE_CURVE_WITH_KNOTS ( ( 3, 2, 2, 2, 3 ),
 ( 0.8958333333333333703, 0.9027777777777777901, 0.9166666666666666297, 0.9305555555555555802, 0.9375000000000000000 ),
 .UNSPECIFIED. ) 
 CURVE ( )  GEOMETRIC_REPRESENTATION_ITEM ( )  RATIONAL_B_SPLINE_CURVE ( ( 0.9330127018922192983, 0.9330127018922198534, 1.000000000000000000, 0.8660254037844387076, 1.000000000000000000, 0.8660254037844387076, 1.000000000000000000, 0.9330127018922194093, 0.9330127018922194093 ) ) 
 REPRESENTATION_ITEM ( '' )  );
#1723=CARTESIAN_POINT ( 'NONE',  ( -1.406733260263382856, -27.42633545031536713, -5.250000000000006217 ) ) ;
#1728=CARTESIAN_POINT ( 'NONE',  ( 2.625000000000000444, -27.70833333333333215, -4.546633369868303021 ) ) ;
#1730=EDGE_CURVE ( 'NONE', #813, #2168, #7834, .T. ) ;
#1731=ORIENTED_EDGE ( 'NONE', *, *, #222, .F. ) ;
#1734=CARTESIAN_POINT ( 'NONE',  ( -2.557341765625002594, -28.44270833367473017, 4.429445870380399164 ) ) ;
#1738=CARTESIAN_POINT ( 'NONE',  ( 0.000000000000000000, -30.00000000000000000, 5.250000000000000000 ) ) ;
#1739=CARTESIAN_POINT ( 'NONE',  ( -5.114683531250000748, -28.79687500034139802, -6.263680815196995234E-16 ) ) ;
#1740=CARTESIAN_POINT ( 'NONE',  ( 2.300847884672513123E-14, -28.21875000068279604, -5.250000000000000000 ) ) ;
#1742=CARTESIAN_POINT ( 'NONE',  ( 6.972266317189433020E-16, -29.93749999999999645, -5.249999999999999112 ) ) ;
#1743=CARTESIAN_POINT ( 'NONE',  ( -5.114683531249999859, -27.75520833367473017, -2.952963913586935440 ) ) ;
#1744=ORIENTED_EDGE ( 'NONE', *, *, #3503, .T. ) ;
#1750=DIRECTION ( 'NONE',  ( 0.000000000000000000, 0.000000000000000000, 1.000000000000000000 ) ) ;
#1753=CARTESIAN_POINT ( 'NONE',  ( -1.406733260263395735, -29.82366454968462932, 5.250000000000000000 ) ) ;
#1754=CARTESIAN_POINT ( 'NONE',  ( -5.250000000000000000, -27.90625000068279604, -6.429395695523604153E-16 ) ) ;
#1755=PRODUCT_DEFINITION_FORMATION_WITH_SPECIFIED_SOURCE ( 'ANY', '', #4597, .NOT_KNOWN. ) ;
#1761=ADVANCED_FACE ( 'NONE', ( #3408 ), #608, .T. ) ;
#1762=EDGE_CURVE ( 'NONE', #7067, #8842, #6237, .T. ) ;
#1767=CARTESIAN_POINT ( 'NONE',  ( 5.114683531249998971, -29.63020833367473017, 2.952963913586936329 ) ) ;
#1775=ORIENTED_EDGE ( 'NONE', *, *, #2638, .T. ) ;
#1776=CARTESIAN_POINT ( 'NONE',  ( 3.712013335537174572E-16, -28.43750000000000000, -6.062177826491070398 ) ) ;
#1777=AXIS2_PLACEMENT_3D ( 'NONE', #4129, #3393, #7622 ) ;
#1779=( BOUNDED_CURVE ( )  B_SPLINE_CURVE ( 2, ( #4094, #556, #3399, #6228, #2884, #4315, #1426, #1610, #4449 ),
 .UNSPECIFIED., .F., .F. ) 
 B_SPLINE_CURVE_WITH_KNOTS ( ( 3, 2, 2, 2, 3 ),
 ( 0.7291666666666667407, 0.7361111111111111605, 0.7500000000000000000, 0.7638888888888888395, 0.7708333333333332593 ),
 .UNSPECIFIED. ) 
 CURVE ( )  GEOMETRIC_REPRESENTATION_ITEM ( )  RATIONAL_B_SPLINE_CURVE ( ( 0.9330127018922192983, 0.9330127018922198534, 1.000000000000000000, 0.8660254037844387076, 1.000000000000000000, 0.8660254037844387076, 1.000000000000000000, 0.9330127018922198534, 0.9330127018922192983 ) ) 
 REPRESENTATION_ITEM ( '' )  );
#1780=ORIENTED_EDGE ( 'NONE', *, *, #4907, .F. ) ;
#1784=CARTESIAN_POINT ( 'NONE',  ( -1.084901341431563726E-15, -29.42187500034139447, 5.905927827173866440 ) ) ;
#1787=CARTESIAN_POINT ( 'NONE',  ( 6.972266317189433020E-16, -28.46875000068279959, -5.249999999999999112 ) ) ;
#1788=CARTESIAN_POINT ( 'NONE',  ( 2.300847884672513123E-14, -28.18750000000000000, -5.250000000000000000 ) ) ;
#1789=CARTESIAN_POINT ( 'NONE',  ( 3.616337804771879580E-16, -28.10937500034140157, -5.905927827173866440 ) ) ;
#1790=VECTOR ( 'NONE', #7690, 1000.000000000000000 ) ;
#1792=CARTESIAN_POINT ( 'NONE',  ( 3.616337804771879580E-16, -27.29687500034139802, -5.905927827173866440 ) ) ;
#1794=EDGE_CURVE ( 'NONE', #1056, #8492, #6936, .T. ) ;
#1797=CARTESIAN_POINT ( 'NONE',  ( 1.406733260263394625, -29.94866454968462577, -5.250000000000000000 ) ) ;
#1799=ORIENTED_EDGE ( 'NONE', *, *, #6925, .T. ) ;
#1802=CARTESIAN_POINT ( 'NONE',  ( 2.625000000000000444, -27.48958333401612819, -4.546633369868303021 ) ) ;
#1806=ORIENTED_EDGE ( 'NONE', *, *, #6793, .F. ) ;
#1810=CARTESIAN_POINT ( 'NONE',  ( 2.300847884672513123E-14, -28.18750000000000000, -5.250000000000000000 ) ) ;
#1814=CARTESIAN_POINT ( 'NONE',  ( 2.557341765625000818, -29.81770833367473372, -4.429445870380400052 ) ) ;
#1823=CARTESIAN_POINT ( 'NONE',  ( 5.250000000000000000, -27.97916666666666430, -3.031088913245534755 ) ) ;
#1824=FACE_OUTER_BOUND ( 'NONE', #8062, .T. ) ;
#1826=ORIENTED_EDGE ( 'NONE', *, *, #6824, .F. ) ;
#1832=CARTESIAN_POINT ( 'NONE',  ( 5.114683531250000748, -28.60937500034139802, 0.000000000000000000 ) ) ;
#1836=CARTESIAN_POINT ( 'NONE',  ( -5.114683531250000748, -29.27604166700806232, 2.952963913586931888 ) ) ;
#1838=ADVANCED_FACE ( 'NONE', ( #1824 ), #564, .T. ) ;
#1842=CARTESIAN_POINT ( 'NONE',  ( 5.114683531249999859, -27.33854166700806232, -2.952963913586932776 ) ) ;
#1849=AXIS2_PLACEMENT_3D ( 'NONE', #1507, #3100, #159 ) ;
#1855=CARTESIAN_POINT ( 'NONE',  ( 2.624999999999996891, -28.32291666734946389, 4.546633369868304797 ) ) ;
#1859=EDGE_CURVE ( 'NONE', #3172, #2054, #418, .T. ) ;
#1862=DIRECTION ( 'NONE',  ( 1.000000000000000000, 0.000000000000000000, 0.000000000000000000 ) ) ;
#1865=CARTESIAN_POINT ( 'NONE',  ( 5.249999999999997335, -28.27083333333332860, 3.031088913245538308 ) ) ;
#1866=CARTESIAN_POINT ( 'NONE',  ( 1.406733260263405061, -27.97991455036742181, -5.249999999999994671 ) ) ;
#1873=DIRECTION ( 'NONE',  ( 0.000000000000000000, 1.000000000000000000, 0.000000000000000000 ) ) ;
#1876=EDGE_LOOP ( 'NONE', ( #7403, #4254, #2030, #5838 ) ) ;
#1879=CARTESIAN_POINT ( 'NONE',  ( 2.557341765624996821, -26.96354166700806232, 4.429445870380401828 ) ) ;
#1880=VERTEX_POINT ( 'NONE', #2710 ) ;
#1883=EDGE_LOOP ( 'NONE', ( #4980, #2956, #8311, #3672 ) ) ;
#1884=CARTESIAN_POINT ( 'NONE',  ( -2.557341765624999042, -29.27604166700806232, -4.429445870380400052 ) ) ;
#1887=CARTESIAN_POINT ( 'NONE',  ( -2.557341765625002594, -27.75520833367473017, 4.429445870380399164 ) ) ;
#1890=CARTESIAN_POINT ( 'NONE',  ( -5.114683531250000748, -26.98437500034139802, -6.263680815196995234E-16 ) ) ;
#1891=CARTESIAN_POINT ( 'NONE',  ( -5.114683531250000748, -29.27604166700806232, 2.952963913586931888 ) ) ;
#1897=ORIENTED_EDGE ( 'NONE', *, *, #7817, .F. ) ;
#1898=CARTESIAN_POINT ( 'NONE',  ( 5.249999999999997335, -29.30208333401613174, 3.031088913245538308 ) ) ;
#1899=CARTESIAN_POINT ( 'NONE',  ( 5.249999999999999112, -27.55208333401613174, 3.031088913245538308 ) ) ;
#1907=DIRECTION ( 'NONE',  ( 0.000000000000000000, 1.000000000000000000, 0.000000000000000000 ) ) ;
#1919=ORIENTED_EDGE ( 'NONE', *, *, #7197, .F. ) ;
#1926=VECTOR ( 'NONE', #6086, 1000.000000000000000 ) ;
#1927=CARTESIAN_POINT ( 'NONE',  ( 2.557341765625000818, -28.56770833367473017, -4.429445870380400052 ) ) ;
#1929=DIRECTION ( 'NONE',  ( 0.000000000000000000, 1.000000000000000000, 0.000000000000000000 ) ) ;
#1930=CARTESIAN_POINT ( 'NONE',  ( -1.084901341431563923E-15, -26.98437500034139802, 5.905927827173866440 ) ) ;
#1932=CARTESIAN_POINT ( 'NONE',  ( -5.114683531250000748, -27.23437500034139802, -6.263680815196995234E-16 ) ) ;
#1933=AXIS2_PLACEMENT_3D ( 'NONE', #8132, #6540, #1008 ) ;
#1934=CARTESIAN_POINT ( 'NONE',  ( 5.250000000000000000, -27.00000000000000000, 0.000000000000000000 ) ) ;
#1935=CARTESIAN_POINT ( 'NONE',  ( 5.114683531249998971, -28.44270833367473017, 2.952963913586936329 ) ) ;
#1936=DIRECTION ( 'NONE',  ( 0.000000000000000000, 1.000000000000000000, 0.000000000000000000 ) ) ;
#1938=DIRECTION ( 'NONE',  ( 0.000000000000000000, -0.000000000000000000, 1.000000000000000000 ) ) ;
#1945=CARTESIAN_POINT ( 'NONE',  ( -1.113604000661152470E-15, -28.59375000068279604, 6.062177826491070398 ) ) ;
#1947=ORIENTED_EDGE ( 'NONE', *, *, #7078, .F. ) ;
#1953=ADVANCED_FACE ( 'NONE', ( #6094 ), #2666, .F. ) ;
#1954=FACE_OUTER_BOUND ( 'NONE', #5271, .T. ) ;
#1969=CARTESIAN_POINT ( 'NONE',  ( 5.114683531250000748, -27.83854166700806587, -2.952963913586932776 ) ) ;
#1972=CARTESIAN_POINT ( 'NONE',  ( -2.557341765624999042, -27.83854166700806587, -4.429445870380400052 ) ) ;
#1974=CARTESIAN_POINT ( 'NONE',  ( -2.557341765624999042, -29.83854166700806232, -4.429445870380400052 ) ) ;
#1976=CARTESIAN_POINT ( 'NONE',  ( 2.557341765625000818, -28.88020833367473017, -4.429445870380400052 ) ) ;
#1977=CARTESIAN_POINT ( 'NONE',  ( -2.625000000000002220, -28.36458333401612819, 4.546633369868302132 ) ) ;
#1987=CARTESIAN_POINT ( 'NONE',  ( -2.557341765624999042, -29.52604166700806232, -4.429445870380400052 ) ) ;
#1991=AXIS2_PLACEMENT_3D ( 'NONE', #8111, #944, #8759 ) ;
#2000=CARTESIAN_POINT ( 'NONE',  ( -2.557341765624999042, -28.52604166700806587, -4.429445870380400052 ) ) ;
#2005=( BOUNDED_CURVE ( )  B_SPLINE_CURVE ( 2, ( #3831, #5964, #7361, #4431, #5169, #102, #4388, #2953, #1547 ),
 .UNSPECIFIED., .F., .T. ) 
 B_SPLINE_CURVE_WITH_KNOTS ( ( 3, 2, 2, 2, 3 ),
 ( 0.7708333333333332593, 0.7777777777777777901, 0.7916666666666666297, 0.8055555555555555802, 0.8125000000000000000 ),
 .UNSPECIFIED. ) 
 CURVE ( )  GEOMETRIC_REPRESENTATION_ITEM ( )  RATIONAL_B_SPLINE_CURVE ( ( 0.9330127018922192983, 0.9330127018922187432, 1.000000000000000000, 0.8660254037844387076, 1.000000000000000000, 0.8660254037844387076, 1.000000000000000000, 0.9330127018922194093, 0.9330127018922194093 ) ) 
 REPRESENTATION_ITEM ( '' )  );
#2010=CARTESIAN_POINT ( 'NONE',  ( 0.000000000000000000, -30.00000000000000000, 0.000000000000000000 ) ) ;
#2014=CARTESIAN_POINT ( 'NONE',  ( -5.114683531250001636, -27.96354166700806587, 2.952963913586931444 ) ) ;
#2016=CARTESIAN_POINT ( 'NONE',  ( -1.084901341431563923E-15, -27.98437500034139802, 5.905927827173866440 ) ) ;
#2019=CARTESIAN_POINT ( 'NONE',  ( 3.616337804771879580E-16, -28.60937500034139802, -5.905927827173866440 ) ) ;
#2020=CARTESIAN_POINT ( 'NONE',  ( -5.114683531249999859, -28.56770833367473017, -2.952963913586935440 ) ) ;
#2030=ORIENTED_EDGE ( 'NONE', *, *, #7078, .T. ) ;
#2031=CARTESIAN_POINT ( 'NONE',  ( 9.180150650966086169E-15, -28.81249999999999645, 5.249999999999999112 ) ) ;
#2032=CARTESIAN_POINT ( 'NONE',  ( -2.557341765625002594, -29.44270833367473017, 4.429445870380399164 ) ) ;
#2041=CARTESIAN_POINT ( 'NONE',  ( -5.114683531249999859, -28.00520833367473017, -2.952963913586935440 ) ) ;
#2044=EDGE_CURVE ( 'NONE', #7888, #784, #2073, .T. ) ;
#2046=CARTESIAN_POINT ( 'NONE',  ( -5.250000000000000000, -28.15625000068279604, -6.429395695523604153E-16 ) ) ;
#2048=ADVANCED_FACE ( 'NONE', ( #5666, #2848 ), #4235, .F. ) ;
#2051=CARTESIAN_POINT ( 'NONE',  ( 2.624999999999996891, -27.29166666666666430, 4.546633369868304797 ) ) ;
#2054=VERTEX_POINT ( 'NONE', #2139 ) ;
#2056=CARTESIAN_POINT ( 'NONE',  ( 2.557341765624996821, -27.15104166700806587, 4.429445870380401828 ) ) ;
#2058=CARTESIAN_POINT ( 'NONE',  ( 2.557341765625000818, -27.63020833367473017, -4.429445870380400052 ) ) ;
#2059=CARTESIAN_POINT ( 'NONE',  ( -5.114683531250000748, -28.56770833367473017, -2.952963913586935440 ) ) ;
#2060=LINE ( 'NONE', #2770, #1790 ) ;
#2061=CARTESIAN_POINT ( 'NONE',  ( -5.114683531250000748, -29.54687500034139802, -6.263680815196995234E-16 ) ) ;
#2062=CARTESIAN_POINT ( 'NONE',  ( 9.180150650966086169E-15, -28.34375000068279604, 5.250000000000000000 ) ) ;
#2064=DIRECTION ( 'NONE',  ( 0.000000000000000000, 1.000000000000000000, 0.000000000000000000 ) ) ;
#2071=CARTESIAN_POINT ( 'NONE',  ( 2.557341765625000818, -29.56770833367473017, -4.429445870380400052 ) ) ;
#2073=( BOUNDED_CURVE ( )  B_SPLINE_CURVE ( 2, ( #4322, #4876, #2051, #2353, #7724, #2180, #2892, #8595, #7815 ),
 .UNSPECIFIED., .F., .T. ) 
 B_SPLINE_CURVE_WITH_KNOTS ( ( 3, 2, 2, 2, 3 ),
 ( 0.8958333333333333703, 0.9027777777777777901, 0.9166666666666666297, 0.9305555555555555802, 0.9375000000000000000 ),
 .UNSPECIFIED. ) 
 CURVE ( )  GEOMETRIC_REPRESENTATION_ITEM ( )  RATIONAL_B_SPLINE_CURVE ( ( 0.9330127018922192983, 0.9330127018922198534, 1.000000000000000000, 0.8660254037844387076, 1.000000000000000000, 0.8660254037844387076, 1.000000000000000000, 0.9330127018922194093, 0.9330127018922194093 ) ) 
 REPRESENTATION_ITEM ( '' )  );
#2074=VERTEX_POINT ( 'NONE', #2226 ) ;
#2079=AXIS2_PLACEMENT_3D ( 'NONE', #1001, #1561, #6628 ) ;
#2080=ORIENTED_EDGE ( 'NONE', *, *, #5233, .F. ) ;
#2081=CARTESIAN_POINT ( 'NONE',  ( -1.406733260263395735, -27.57366454968463287, 5.250000000000000000 ) ) ;
#2086=CARTESIAN_POINT ( 'NONE',  ( 5.114683531249999859, -29.08854166700806942, -2.952963913586932776 ) ) ;
#2090=EDGE_CURVE ( 'NONE', #7322, #874, #8621, .T. ) ;
#2097=CARTESIAN_POINT ( 'NONE',  ( 6.972266317189433020E-16, -26.96875000068279249, -5.250000000000000000 ) ) ;
#2101=CARTESIAN_POINT ( 'NONE',  ( -2.557341765625002594, -27.44270833367473017, 4.429445870380399164 ) ) ;
#2103=CARTESIAN_POINT ( 'NONE',  ( 5.250000000000000000, -28.72916666666666785, -3.031088913245534755 ) ) ;
#2105=CARTESIAN_POINT ( 'NONE',  ( -5.114683531250000748, -29.29687500034139802, -6.263680815196995234E-16 ) ) ;
#2106=CARTESIAN_POINT ( 'NONE',  ( 2.557341765624996821, -27.21354166700806587, 4.429445870380401828 ) ) ;
#2110=CARTESIAN_POINT ( 'NONE',  ( 1.406733260263393070, -29.47991455036742181, -5.250000000000000888 ) ) ;
#2111=CARTESIAN_POINT ( 'NONE',  ( 2.624999999999996891, -28.54166666666666785, 4.546633369868304797 ) ) ;
#2114=EDGE_LOOP ( 'NONE', ( #6518, #6060, #376, #5968 ) ) ;
#2116=CARTESIAN_POINT ( 'NONE',  ( -2.624999999999998668, -27.19791666734946389, -4.546633369868303021 ) ) ;
#2121=CARTESIAN_POINT ( 'NONE',  ( 0.000000000000000000, 75.00000000000000000, 0.000000000000000000 ) ) ;
#2126=( BOUNDED_CURVE ( )  B_SPLINE_CURVE ( 2, ( #8324, #2562, #9009, #9057, #8372, #2654, #7485, #1866, #7580 ),
 .UNSPECIFIED., .F., .F. ) 
 B_SPLINE_CURVE_WITH_KNOTS ( ( 3, 2, 2, 2, 3 ),
 ( 0.5625000000000000000, 0.5694444444444444198, 0.5833333333333333703, 0.5972222222222222099, 0.6041666666666666297 ),
 .UNSPECIFIED. ) 
 CURVE ( )  GEOMETRIC_REPRESENTATION_ITEM ( )  RATIONAL_B_SPLINE_CURVE ( ( 0.9330127018922194093, 0.9330127018922194093, 1.000000000000000000, 0.8660254037844387076, 1.000000000000000000, 0.8660254037844387076, 1.000000000000000000, 0.9330127018922198534, 0.9330127018922192983 ) ) 
 REPRESENTATION_ITEM ( '' )  );
#2129=CARTESIAN_POINT ( 'NONE',  ( -1.084901341431563923E-15, -28.42187500034139802, 5.905927827173866440 ) ) ;
#2131=MANIFOLD_SOLID_BREP ( 'Thread1', #7871 ) ;
#2135=FACE_OUTER_BOUND ( 'NONE', #5491, .T. ) ;
#2138=VECTOR ( 'NONE', #7889, 1000.000000000000000 ) ;
#2139=CARTESIAN_POINT ( 'NONE',  ( -1.975475456537005874E-15, -28.31249999999999645, 5.249999999999999112 ) ) ;
#2140=ADVANCED_FACE ( 'NONE', ( #5620, #83 ), #8469, .F. ) ;
#2141=CARTESIAN_POINT ( 'NONE',  ( -5.250000000000000000, -27.87500000000000000, -6.429395695523604153E-16 ) ) ;
#2145=ORIENTED_EDGE ( 'NONE', *, *, #4082, .T. ) ;
#2146=CARTESIAN_POINT ( 'NONE',  ( 5.114683531249998971, -27.38020833367473372, 2.952963913586936329 ) ) ;
#2149=CARTESIAN_POINT ( 'NONE',  ( -5.250000000000000888, -29.35416666666666430, 3.031088913245532979 ) ) ;
#2151=CARTESIAN_POINT ( 'NONE',  ( 5.114683531250000748, -28.67187500034139802, 0.000000000000000000 ) ) ;
#2153=CARTESIAN_POINT ( 'NONE',  ( 5.114683531249998971, -28.19270833367473372, 2.952963913586936329 ) ) ;
#2157=CARTESIAN_POINT ( 'NONE',  ( 9.180150650966086169E-15, -28.56249999999999645, 5.250000000000000000 ) ) ;
#2162=CARTESIAN_POINT ( 'NONE',  ( -5.250000000000000000, -26.92708333401612819, -3.031088913245536531 ) ) ;
#2168=VERTEX_POINT ( 'NONE', #8369 ) ;
#2172=CARTESIAN_POINT ( 'NONE',  ( 2.557341765624996821, -28.15104166700806587, 4.429445870380401828 ) ) ;
#2173=FACE_OUTER_BOUND ( 'NONE', #8068, .T. ) ;
#2175=CARTESIAN_POINT ( 'NONE',  ( -2.625000000000002220, -28.86458333401612819, 4.546633369868302132 ) ) ;
#2180=CARTESIAN_POINT ( 'NONE',  ( 5.249999999999999112, -27.22916666666666430, -3.031088913245534755 ) ) ;
#2181=CARTESIAN_POINT ( 'NONE',  ( 0.000000000000000000, -30.00000000000000000, 5.250000000000000000 ) ) ;
#2182=ADVANCED_FACE ( 'NONE', ( #6075, #4090 ), #7668, .T. ) ;
#2185=ORIENTED_EDGE ( 'NONE', *, *, #5655, .T. ) ;
#2186=DIRECTION ( 'NONE',  ( 0.000000000000000000, 0.000000000000000000, 1.000000000000000000 ) ) ;
#2189=CARTESIAN_POINT ( 'NONE',  ( 2.625000000000000444, -29.70833333333333215, -4.546633369868303021 ) ) ;
#2190=FACE_OUTER_BOUND ( 'NONE', #1371, .T. ) ;
#2192=CARTESIAN_POINT ( 'NONE',  ( 2.557341765624996821, -27.46354166700806587, 4.429445870380401828 ) ) ;
#2193=EDGE_CURVE ( 'NONE', #8808, #3057, #763, .T. ) ;
#2195=CARTESIAN_POINT ( 'NONE',  ( 5.114683531249999859, -27.65104166700806232, -2.952963913586932776 ) ) ;
#2196=DIRECTION ( 'NONE',  ( 0.000000000000000000, 1.000000000000000000, 0.000000000000000000 ) ) ;
#2200=CARTESIAN_POINT ( 'NONE',  ( 5.114683531249999859, -29.65104166700806232, -2.952963913586932776 ) ) ;
#2204=CARTESIAN_POINT ( 'NONE',  ( 5.250000000000000000, -27.99999999999999645, 0.000000000000000000 ) ) ;
#2205=CARTESIAN_POINT ( 'NONE',  ( -5.114683531250000748, -27.96354166700806587, 2.952963913586931888 ) ) ;
#2208=DIRECTION ( 'NONE',  ( 0.000000000000000000, 0.000000000000000000, 1.000000000000000000 ) ) ;
#2213=CARTESIAN_POINT ( 'NONE',  ( -5.250000000000000000, -27.62500000000000000, -6.429395695523604153E-16 ) ) ;
#2217=CARTESIAN_POINT ( 'NONE',  ( -5.114683531250000748, -27.73437500034139802, -6.263680815196995234E-16 ) ) ;
#2225=CIRCLE ( 'NONE', #7429, 2.750000000000000000 ) ;
#2226=CARTESIAN_POINT ( 'NONE',  ( 0.000000000000000000, -9.000000000000001776, 5.250000000000000000 ) ) ;
#2227=CARTESIAN_POINT ( 'NONE',  ( -5.250000000000000000, -26.90625000068279604, -6.429395695523604153E-16 ) ) ;
#2229=DIRECTION ( 'NONE',  ( 0.000000000000000000, 0.000000000000000000, 1.000000000000000000 ) ) ;
#2230=ORIENTED_EDGE ( 'NONE', *, *, #6137, .T. ) ;
#2235=VECTOR ( 'NONE', #6110, 1000.000000000000000 ) ;
#2237=CARTESIAN_POINT ( 'NONE',  ( -1.113604000661152470E-15, -29.06250000000000000, 6.062177826491070398 ) ) ;
#2239=( BOUNDED_CURVE ( )  B_SPLINE_CURVE ( 2, ( #727, #2886, #1427, #683, #6948, #8547, #2175, #9148, #4955 ),
 .UNSPECIFIED., .F., .F. ) 
 B_SPLINE_CURVE_WITH_KNOTS ( ( 3, 2, 2, 2, 3 ),
 ( 0.2708333333333333148, 0.2777777777777777901, 0.2916666666666666852, 0.3055555555555555802, 0.3125000000000000000 ),
 .UNSPECIFIED. ) 
 CURVE ( )  GEOMETRIC_REPRESENTATION_ITEM ( )  RATIONAL_B_SPLINE_CURVE ( ( 0.9330127018922194093, 0.9330127018922190762, 1.000000000000000000, 0.8660254037844387076, 1.000000000000000000, 0.8660254037844387076, 1.000000000000000000, 0.9330127018922194093, 0.9330127018922194093 ) ) 
 REPRESENTATION_ITEM ( '' )  );
#2240=CARTESIAN_POINT ( 'NONE',  ( -5.114683531250000748, -27.29687500034139802, -6.263680815196995234E-16 ) ) ;
#2243=CARTESIAN_POINT ( 'NONE',  ( -5.114683531250000748, -28.04687500034139802, -6.263680815196995234E-16 ) ) ;
#2247=CARTESIAN_POINT ( 'NONE',  ( -1.084901341431563923E-15, -29.48437500034139802, 5.905927827173866440 ) ) ;
#2252=CARTESIAN_POINT ( 'NONE',  ( -1.084901341431563923E-15, -27.92187500034139802, 5.905927827173866440 ) ) ;
#2256=LINE ( 'NONE', #3700, #3036 ) ;
#2262=CARTESIAN_POINT ( 'NONE',  ( 3.712013335537174572E-16, -29.46875000068279604, -6.062177826491070398 ) ) ;
#2265=CARTESIAN_POINT ( 'NONE',  ( -5.114683531249999859, -27.25520833367473017, -2.952963913586935440 ) ) ;
#2285=CARTESIAN_POINT ( 'NONE',  ( 5.250000000000000000, -29.75000000000000000, 0.000000000000000000 ) ) ;
#2287=CARTESIAN_POINT ( 'NONE',  ( -1.084901341431563726E-15, -27.48437500034139802, 5.905927827173866440 ) ) ;
#2289=CARTESIAN_POINT ( 'NONE',  ( -5.114683531250000748, -27.29687500034139802, -6.263680815196995234E-16 ) ) ;
#2290=CARTESIAN_POINT ( 'NONE',  ( 0.000000000000000000, -30.00000000000000000, 0.000000000000000000 ) ) ;
#2295=CARTESIAN_POINT ( 'NONE',  ( 2.557341765625000818, -29.88020833367473372, -4.429445870380400052 ) ) ;
#2298=EDGE_LOOP ( 'NONE', ( #5873, #4439, #7699, #7334 ) ) ;
#2301=CARTESIAN_POINT ( 'NONE',  ( 3.616337804771879580E-16, -29.04687500034139802, -5.905927827173866440 ) ) ;
#2303=ORIENTED_EDGE ( 'NONE', *, *, #1165, .F. ) ;
#2305=CARTESIAN_POINT ( 'NONE',  ( 0.000000000000000000, -30.00000000000000000, 0.000000000000000000 ) ) ;
#2308=CARTESIAN_POINT ( 'NONE',  ( -5.250000000000000888, -29.10416666666666785, 3.031088913245533423 ) ) ;
#2309=ORIENTED_EDGE ( 'NONE', *, *, #5158, .T. ) ;
#2311=LINE ( 'NONE', #165, #6391 ) ;
#2313=CARTESIAN_POINT ( 'NONE',  ( 2.557341765624996821, -27.90104166700806587, 4.429445870380401828 ) ) ;
#2322=DIRECTION ( 'NONE',  ( 0.000000000000000000, 1.000000000000000000, 0.000000000000000000 ) ) ;
#2323=ORIENTED_EDGE ( 'NONE', *, *, #8402, .T. ) ;
#2325=EDGE_CURVE ( 'NONE', #8116, #4614, #3674, .T. ) ;
#2329=CARTESIAN_POINT ( 'NONE',  ( 5.114683531250000748, -26.85937500034139802, 0.000000000000000000 ) ) ;
#2332=CARTESIAN_POINT ( 'NONE',  ( -5.250000000000000000, -27.39583333333332860, -3.031088913245536531 ) ) ;
#2333=CARTESIAN_POINT ( 'NONE',  ( -1.084901341431563726E-15, -27.98437500034139802, 5.905927827173866440 ) ) ;
#2338=CARTESIAN_POINT ( 'NONE',  ( 6.972266317189433020E-16, -28.68749999999999645, -5.250000000000000000 ) ) ;
#2339=DIRECTION ( 'NONE',  ( 1.000000000000000000, 0.000000000000000000, 0.000000000000000000 ) ) ;
#2342=ORIENTED_EDGE ( 'NONE', *, *, #3349, .T. ) ;
#2344=CARTESIAN_POINT ( 'NONE',  ( 2.624999999999996891, -28.04166666666666785, 4.546633369868304797 ) ) ;
#2345=CARTESIAN_POINT ( 'NONE',  ( -2.557341765625002594, -27.94270833367473017, 4.429445870380399164 ) ) ;
#2346=( BOUNDED_CURVE ( )  B_SPLINE_CURVE ( 2, ( #3197, #6018, #393, #1797, #4767 ),
 .UNSPECIFIED., .F., .F. ) 
 B_SPLINE_CURVE_WITH_KNOTS ( ( 3, 2, 3 ),
 ( 0.000000000000000000, 0.01388888888888888812, 0.02083333333333333218 ),
 .UNSPECIFIED. ) 
 CURVE ( )  GEOMETRIC_REPRESENTATION_ITEM ( )  RATIONAL_B_SPLINE_CURVE ( ( 1.000000000000000000, 0.8660254037844387076, 1.000000000000000000, 0.9330127018922194093, 0.9330127018922194093 ) ) 
 REPRESENTATION_ITEM ( '' )  );
#2348=CARTESIAN_POINT ( 'NONE',  ( 2.033577675846918216E-14, -26.84375000068279959, 5.250000000000000888 ) ) ;
#2353=CARTESIAN_POINT ( 'NONE',  ( 5.249999999999997335, -27.27083333333332860, 3.031088913245538308 ) ) ;
#2356=CARTESIAN_POINT ( 'NONE',  ( -2.625000000000002220, -29.11458333401613174, 4.546633369868302132 ) ) ;
#2358=CARTESIAN_POINT ( 'NONE',  ( -2.557341765625002594, -29.75520833367473017, 4.429445870380399164 ) ) ;
#2363=DIRECTION ( 'NONE',  ( 0.000000000000000000, 1.000000000000000000, 0.000000000000000000 ) ) ;
#2372=( BOUNDED_CURVE ( )  B_SPLINE_CURVE ( 2, ( #5337, #363, #8187, #4647, #6782, #7488, #6640, #3122, #3955 ),
 .UNSPECIFIED., .F., .T. ) 
 B_SPLINE_CURVE_WITH_KNOTS ( ( 3, 2, 2, 2, 3 ),
 ( 0.7291666666666667407, 0.7361111111111111605, 0.7500000000000000000, 0.7638888888888888395, 0.7708333333333332593 ),
 .UNSPECIFIED. ) 
 CURVE ( )  GEOMETRIC_REPRESENTATION_ITEM ( )  RATIONAL_B_SPLINE_CURVE ( ( 0.9330127018922192983, 0.9330127018922198534, 1.000000000000000000, 0.8660254037844387076, 1.000000000000000000, 0.8660254037844387076, 1.000000000000000000, 0.9330127018922198534, 0.9330127018922192983 ) ) 
 REPRESENTATION_ITEM ( '' )  );
#2376=EDGE_LOOP ( 'NONE', ( #3934, #6046, #8764, #5352 ) ) ;
#2380=CARTESIAN_POINT ( 'NONE',  ( 3.712013335537174572E-16, -27.18750000000000000, -6.062177826491070398 ) ) ;
#2382=CARTESIAN_POINT ( 'NONE',  ( 5.114683531250000748, -28.15104166700806587, -2.952963913586932776 ) ) ;
#2385=CARTESIAN_POINT ( 'NONE',  ( -5.114683531250000748, -29.73437500034139802, -6.263680815196995234E-16 ) ) ;
#2387=CARTESIAN_POINT ( 'NONE',  ( 5.114683531250000748, -29.89062500034139802, 0.000000000000000000 ) ) ;
#2388=CARTESIAN_POINT ( 'NONE',  ( 5.250000000000000000, -28.74999999999999645, 0.000000000000000000 ) ) ;
#2389=CARTESIAN_POINT ( 'NONE',  ( 3.616337804771879580E-16, -29.10937500034139447, -5.905927827173866440 ) ) ;
#2390=CARTESIAN_POINT ( 'NONE',  ( 1.406733260263397289, -28.33258545099817027, 5.249999999999997335 ) ) ;
#2394=CARTESIAN_POINT ( 'NONE',  ( -5.114683531250000748, -28.71354166700806587, 2.952963913586931888 ) ) ;
#2396=DIRECTION ( 'NONE',  ( 0.000000000000000000, 1.000000000000000000, 0.000000000000000000 ) ) ;
#2403=CARTESIAN_POINT ( 'NONE',  ( -5.250000000000000000, -29.17708333401612819, -3.031088913245536531 ) ) ;
#2405=CARTESIAN_POINT ( 'NONE',  ( 2.557341765625000818, -27.06770833367473017, -4.429445870380400052 ) ) ;
#2406=EDGE_LOOP ( 'NONE', ( #260, #3747, #8339, #5465 ) ) ;
#2409=LINE ( 'NONE', #7337, #2824 ) ;
#2410=EDGE_CURVE ( 'NONE', #977, #3365, #4358, .T. ) ;
#2412=CARTESIAN_POINT ( 'NONE',  ( 0.000000000000000000, -30.00000000000000000, 0.000000000000000000 ) ) ;
#2416=DIRECTION ( 'NONE',  ( 1.000000000000000000, 0.000000000000000000, 0.000000000000000000 ) ) ;
#2421=ORIENTED_EDGE ( 'NONE', *, *, #5655, .F. ) ;
#2425=ORIENTED_EDGE ( 'NONE', *, *, #362, .T. ) ;
#2426=CARTESIAN_POINT ( 'NONE',  ( -2.625000000000002220, -28.33333333333333215, 4.546633369868302132 ) ) ;
#2429=CARTESIAN_POINT ( 'NONE',  ( 5.114683531249998971, -26.94270833367473372, 2.952963913586936329 ) ) ;
#2432=SURFACE_SIDE_STYLE ('',( #8055 ) ) ;
#2435=CARTESIAN_POINT ( 'NONE',  ( 3.616337804771879580E-16, -28.54687500034139802, -5.905927827173866440 ) ) ;
#2437=CARTESIAN_POINT ( 'NONE',  ( 5.114683531250000748, -26.92187500034139802, 0.000000000000000000 ) ) ;
#2439=CARTESIAN_POINT ( 'NONE',  ( 2.557341765625000818, -29.38020833367473017, -4.429445870380400052 ) ) ;
#2444=CARTESIAN_POINT ( 'NONE',  ( -5.114683531249999859, -27.25520833367473017, -2.952963913586935440 ) ) ;
#2446=EDGE_LOOP ( 'NONE', ( #6124, #8578, #8790, #2452 ) ) ;
#2450=CARTESIAN_POINT ( 'NONE',  ( 2.300847884672513123E-14, -28.43750000000000000, -5.250000000000000000 ) ) ;
#2452=ORIENTED_EDGE ( 'NONE', *, *, #3497, .F. ) ;
#2454=CARTESIAN_POINT ( 'NONE',  ( 3.712013335537174572E-16, -29.71875000068279604, -6.062177826491070398 ) ) ;
#2457=ORIENTED_EDGE ( 'NONE', *, *, #8536, .T. ) ;
#2469=CARTESIAN_POINT ( 'NONE',  ( -5.250000000000000000, -27.37500000000000000, -6.429395695523604153E-16 ) ) ;
#2473=ORIENTED_EDGE ( 'NONE', *, *, #4027, .F. ) ;
#2474=CARTESIAN_POINT ( 'NONE',  ( 5.250000000000000000, -27.50000000000000000, 0.000000000000000000 ) ) ;
#2477=ORIENTED_EDGE ( 'NONE', *, *, #4082, .F. ) ;
#2480=ORIENTED_EDGE ( 'NONE', *, *, #1050, .F. ) ;
#2481=CARTESIAN_POINT ( 'NONE',  ( -5.114683531250000748, -29.00520833367473017, -2.952963913586935440 ) ) ;
#2483=CARTESIAN_POINT ( 'NONE',  ( 5.249999999999997335, -28.55208333401612819, 3.031088913245538308 ) ) ;
#2485=CARTESIAN_POINT ( 'NONE',  ( 5.114683531250000748, -28.17187500034139447, 0.000000000000000000 ) ) ;
#2486=CARTESIAN_POINT ( 'NONE',  ( 1.406733260263391960, -27.33258545099816672, 5.250000000000000000 ) ) ;
#2488=CARTESIAN_POINT ( 'NONE',  ( 5.249999999999997335, -29.27083333333333570, 3.031088913245538308 ) ) ;
#2489=CARTESIAN_POINT ( 'NONE',  ( 5.114683531250000748, -27.60937500034139802, 0.000000000000000000 ) ) ;
#2496=ORIENTED_EDGE ( 'NONE', *, *, #9064, .T. ) ;
#2498=CARTESIAN_POINT ( 'NONE',  ( -5.250000000000000000, -28.17708333401613174, -3.031088913245536531 ) ) ;
#2504=CARTESIAN_POINT ( 'NONE',  ( 0.000000000000000000, -30.00000000000000000, 5.250000000000000000 ) ) ;
#2506=DIRECTION ( 'NONE',  ( 0.000000000000000000, 0.000000000000000000, -1.000000000000000000 ) ) ;
#2509=CARTESIAN_POINT ( 'NONE',  ( -5.114683531250000748, -29.71354166700806232, 2.952963913586931888 ) ) ;
#2511=SHAPE_DEFINITION_REPRESENTATION ( #357, #4551 ) ;
#2515=CARTESIAN_POINT ( 'NONE',  ( 0.000000000000000000, -30.00000000000000000, 0.000000000000000000 ) ) ;
#2519=CARTESIAN_POINT ( 'NONE',  ( 2.625000000000000444, -27.95833333333333215, -4.546633369868303021 ) ) ;
#2520=AXIS2_PLACEMENT_3D ( 'NONE', #2121, #4947, #7803 ) ;
#2523=CARTESIAN_POINT ( 'NONE',  ( -5.114683531250001636, -27.02604166700806587, 2.952963913586931444 ) ) ;
#2528=CARTESIAN_POINT ( 'NONE',  ( 5.114683531250000748, -29.08854166700806942, -2.952963913586932776 ) ) ;
#2533=CARTESIAN_POINT ( 'NONE',  ( 5.114683531249998971, -29.19270833367473017, 2.952963913586936329 ) ) ;
#2536=CARTESIAN_POINT ( 'NONE',  ( 2.033577675846918216E-14, -27.84375000068279959, 5.250000000000000888 ) ) ;
#2537=DIRECTION ( 'NONE',  ( 0.000000000000000000, 1.000000000000000000, 0.000000000000000000 ) ) ;
#2540=ORIENTED_EDGE ( 'NONE', *, *, #4138, .F. ) ;
#2543=CARTESIAN_POINT ( 'NONE',  ( -5.250000000000000000, -28.62499999999999645, -6.429395695523604153E-16 ) ) ;
#2544=DIRECTION ( 'NONE',  ( 0.000000000000000000, 0.000000000000000000, 1.000000000000000000 ) ) ;
#2547=VERTEX_POINT ( 'NONE', #7847 ) ;
#2548=AXIS2_PLACEMENT_3D ( 'NONE', #432, #2537, #8937 ) ;
#2551=CARTESIAN_POINT ( 'NONE',  ( -2.624999999999998668, -28.19791666734946389, -4.546633369868303021 ) ) ;
#2554=ORIENTED_EDGE ( 'NONE', *, *, #3417, .F. ) ;
#2562=CARTESIAN_POINT ( 'NONE',  ( 1.406733260263391960, -28.08258545099816672, 5.250000000000000000 ) ) ;
#2564=CARTESIAN_POINT ( 'NONE',  ( 5.114683531249998971, -29.38020833367473017, 2.952963913586936329 ) ) ;
#2565=VERTEX_POINT ( 'NONE', #5184 ) ;
#2577=ORIENTED_EDGE ( 'NONE', *, *, #4348, .T. ) ;
#2581=CARTESIAN_POINT ( 'NONE',  ( 5.114683531249998971, -29.13020833367473017, 2.952963913586936329 ) ) ;
#2584=CARTESIAN_POINT ( 'NONE',  ( 5.114683531250000748, -27.42187500034139802, 0.000000000000000000 ) ) ;
#2588=CARTESIAN_POINT ( 'NONE',  ( 1.185285273922203525E-14, -29.18750000000000000, -5.250000000000000000 ) ) ;
#2589=CARTESIAN_POINT ( 'NONE',  ( -1.084901341431563923E-15, -27.42187500034139802, 5.905927827173866440 ) ) ;
#2590=CARTESIAN_POINT ( 'NONE',  ( -5.114683531249999859, -29.31770833367473372, -2.952963913586935440 ) ) ;
#2593=ADVANCED_FACE ( 'NONE', ( #3065 ), #8027, .T. ) ;
#2596=VECTOR ( 'NONE', #3638, 1000.000000000000000 ) ;
#2602=CARTESIAN_POINT ( 'NONE',  ( 5.250000000000000000, -27.53125000068279604, 0.000000000000000000 ) ) ;
#2610=( BOUNDED_CURVE ( )  B_SPLINE_CURVE ( 2, ( #5276, #953, #1702, #8073, #5928, #2308, #4495, #7190, #6625 ),
 .UNSPECIFIED., .F., .F. ) 
 B_SPLINE_CURVE_WITH_KNOTS ( ( 3, 2, 2, 2, 3 ),
 ( 0.2708333333333333148, 0.2777777777777777901, 0.2916666666666666852, 0.3055555555555555802, 0.3125000000000000000 ),
 .UNSPECIFIED. ) 
 CURVE ( )  GEOMETRIC_REPRESENTATION_ITEM ( )  RATIONAL_B_SPLINE_CURVE ( ( 0.9330127018922194093, 0.9330127018922190762, 1.000000000000000000, 0.8660254037844387076, 1.000000000000000000, 0.8660254037844387076, 1.000000000000000000, 0.9330127018922194093, 0.9330127018922194093 ) ) 
 REPRESENTATION_ITEM ( '' )  );
#2622=ORIENTED_EDGE ( 'NONE', *, *, #1762, .F. ) ;
#2623=CARTESIAN_POINT ( 'NONE',  ( -5.250000000000000000, -27.14583333333333570, -3.031088913245536531 ) ) ;
#2630=CARTESIAN_POINT ( 'NONE',  ( -1.084901341431563726E-15, -28.92187500034139447, 5.905927827173866440 ) ) ;
#2632=LINE ( 'NONE', #1738, #6720 ) ;
#2633=CARTESIAN_POINT ( 'NONE',  ( 5.114683531249999859, -27.15104166700806232, -2.952963913586932776 ) ) ;
#2634=CARTESIAN_POINT ( 'NONE',  ( 3.616337804771879580E-16, -27.54687500034140157, -5.905927827173866440 ) ) ;
#2635=DIRECTION ( 'NONE',  ( 0.000000000000000000, 0.000000000000000000, 1.000000000000000000 ) ) ;
#2636=CARTESIAN_POINT ( 'NONE',  ( 3.616337804771879580E-16, -28.85937500034139802, -5.905927827173866440 ) ) ;
#2637=LINE ( 'NONE', #8211, #3853 ) ;
#2638=EDGE_CURVE ( 'NONE', #3248, #4378, #4326, .T. ) ;
#2640=CARTESIAN_POINT ( 'NONE',  ( 6.972266317189433020E-16, -29.21875000068279249, -5.250000000000000000 ) ) ;
#2644=ORIENTED_EDGE ( 'NONE', *, *, #8333, .T. ) ;
#2646=CARTESIAN_POINT ( 'NONE',  ( 2.624999999999996891, -28.57291666734946389, 4.546633369868304797 ) ) ;
#2653=CARTESIAN_POINT ( 'NONE',  ( 1.406733260263391960, -28.30133545031536713, 5.250000000000000000 ) ) ;
#2654=CARTESIAN_POINT ( 'NONE',  ( 5.249999999999999112, -28.01041666734946389, -3.031088913245534755 ) ) ;
#2661=( BOUNDED_CURVE ( )  B_SPLINE_CURVE ( 2, ( #6777, #9052, #403, #6178, #550, #1250, #5328, #6829, #4045 ),
 .UNSPECIFIED., .F., .F. ) 
 B_SPLINE_CURVE_WITH_KNOTS ( ( 3, 2, 2, 2, 3 ),
 ( 0.1458333333333333426, 0.1527777777777777901, 0.1666666666666666574, 0.1805555555555555525, 0.1875000000000000000 ),
 .UNSPECIFIED. ) 
 CURVE ( )  GEOMETRIC_REPRESENTATION_ITEM ( )  RATIONAL_B_SPLINE_CURVE ( ( 0.9330127018922194093, 0.9330127018922194093, 1.000000000000000000, 0.8660254037844387076, 1.000000000000000000, 0.8660254037844387076, 1.000000000000000000, 0.9330127018922194093, 0.9330127018922194093 ) ) 
 REPRESENTATION_ITEM ( '' )  );
#2666=CYLINDRICAL_SURFACE ( 'NONE', #1649, 4.250000000000000000 ) ;
#2672=CARTESIAN_POINT ( 'NONE',  ( 3.616337804771879580E-16, -27.04687500034139802, -5.905927827173866440 ) ) ;
#2674=CARTESIAN_POINT ( 'NONE',  ( -2.557341765625002594, -27.25520833367473017, 4.429445870380399164 ) ) ;
#2675=DIRECTION ( 'NONE',  ( 0.000000000000000000, 1.000000000000000000, 0.000000000000000000 ) ) ;
#2676=CARTESIAN_POINT ( 'NONE',  ( -5.114683531250000748, -29.04687500034139802, -6.263680815196995234E-16 ) ) ;
#2678=CARTESIAN_POINT ( 'NONE',  ( -2.557341765624999042, -29.08854166700806587, -4.429445870380400052 ) ) ;
#2689=DIRECTION ( 'NONE',  ( 0.000000000000000000, 0.000000000000000000, 1.000000000000000000 ) ) ;
#2691=CARTESIAN_POINT ( 'NONE',  ( -2.625000000000002220, -27.61458333401612819, 4.546633369868302132 ) ) ;
#2694=CARTESIAN_POINT ( 'NONE',  ( -1.975475456537005874E-15, -29.56250000000000000, 5.249999999999999112 ) ) ;
#2701=CARTESIAN_POINT ( 'NONE',  ( -5.114683531250000748, -28.21354166700806232, 2.952963913586931888 ) ) ;
#2702=LINE ( 'NONE', #1383, #6416 ) ;
#2709=CARTESIAN_POINT ( 'NONE',  ( 5.249999999999999112, -27.02083333333333570, 3.031088913245538308 ) ) ;
#2710=CARTESIAN_POINT ( 'NONE',  ( -2.324088772396477476E-15, -29.68750000000000000, -5.250000000000000000 ) ) ;
#2711=EDGE_CURVE ( 'NONE', #3105, #8178, #3980, .T. ) ;
#2712=ADVANCED_FACE ( 'NONE', ( #5321 ), #6171, .T. ) ;
#2716=VERTEX_POINT ( 'NONE', #5517 ) ;
#2717=CARTESIAN_POINT ( 'NONE',  ( 2.557341765625000818, -27.56770833367473017, -4.429445870380400052 ) ) ;
#2719=CARTESIAN_POINT ( 'NONE',  ( -2.557341765625002594, -28.00520833367473017, 4.429445870380399164 ) ) ;
#2720=CARTESIAN_POINT ( 'NONE',  ( 0.000000000000000000, -9.000000000000000000, 0.000000000000000000 ) ) ;
#2721=CARTESIAN_POINT ( 'NONE',  ( 2.557341765625000818, -28.63020833367473017, -4.429445870380400052 ) ) ;
#2722=CARTESIAN_POINT ( 'NONE',  ( -2.557341765624999042, -29.33854166700806232, -4.429445870380400052 ) ) ;
#2723=DIRECTION ( 'NONE',  ( 0.000000000000000000, 1.000000000000000000, 0.000000000000000000 ) ) ;
#2735=CARTESIAN_POINT ( 'NONE',  ( -1.113604000661152470E-15, -27.09375000068279604, 6.062177826491070398 ) ) ;
#2749=CARTESIAN_POINT ( 'NONE',  ( -5.114683531250000748, -29.21354166700806587, 2.952963913586931888 ) ) ;
#2764=CARTESIAN_POINT ( 'NONE',  ( -2.557341765624999042, -27.02604166700806232, -4.429445870380400052 ) ) ;
#2766=CARTESIAN_POINT ( 'NONE',  ( -5.114683531250000748, -27.54687500034139802, -6.263680815196995234E-16 ) ) ;
#2767=CARTESIAN_POINT ( 'NONE',  ( 0.000000000000000000, -30.00000000000000000, 0.000000000000000000 ) ) ;
#2769=CARTESIAN_POINT ( 'NONE',  ( -2.557341765624999042, -28.58854166700806587, -4.429445870380400052 ) ) ;
#2770=CARTESIAN_POINT ( 'NONE',  ( 6.429395695523604153E-16, -30.00000000000000000, -5.250000000000000000 ) ) ;
#2771=CARTESIAN_POINT ( 'NONE',  ( 2.557341765624996821, -28.46354166700806587, 4.429445870380401828 ) ) ;
#2774=CARTESIAN_POINT ( 'NONE',  ( 6.429395695523604153E-16, -9.999999999999998224, -5.250000000000000000 ) ) ;
#2781=CARTESIAN_POINT ( 'NONE',  ( -5.114683531250000748, -29.71354166700806232, 2.952963913586931888 ) ) ;
#2783=ORIENTED_EDGE ( 'NONE', *, *, #5363, .T. ) ;
#2792=CARTESIAN_POINT ( 'NONE',  ( -2.557341765625002594, -28.19270833367473017, 4.429445870380399164 ) ) ;
#2797=CARTESIAN_POINT ( 'NONE',  ( -1.406733260263395735, -28.10491455036742536, 5.250000000000000000 ) ) ;
#2802=DIRECTION ( 'NONE',  ( 0.000000000000000000, 1.000000000000000000, 0.000000000000000000 ) ) ;
#2807=CARTESIAN_POINT ( 'NONE',  ( 2.557341765624996821, -27.90104166700806587, 4.429445870380401828 ) ) ;
#2809=CARTESIAN_POINT ( 'NONE',  ( -5.250000000000000888, -28.85416666666666785, 3.031088913245532979 ) ) ;
#2811=CARTESIAN_POINT ( 'NONE',  ( -5.114683531250000748, -28.54687500034139802, -6.263680815196995234E-16 ) ) ;
#2813=AXIS2_PLACEMENT_3D ( 'NONE', #5574, #8419, #3666 ) ;
#2814=CARTESIAN_POINT ( 'NONE',  ( 5.114683531249998971, -27.69270833367472662, 2.952963913586936329 ) ) ;
#2815=CARTESIAN_POINT ( 'NONE',  ( 6.972266317189433020E-16, -28.46875000068279959, -5.250000000000000000 ) ) ;
#2824=VECTOR ( 'NONE', #3809, 1000.000000000000114 ) ;
#2826=CARTESIAN_POINT ( 'NONE',  ( -5.114683531250000748, -29.21354166700806587, 2.952963913586931888 ) ) ;
#2827=EDGE_CURVE ( 'NONE', #4261, #5029, #6109, .T. ) ;
#2828=ORIENTED_EDGE ( 'NONE', *, *, #6113, .F. ) ;
#2829=VECTOR ( 'NONE', #7877, 1000.000000000000000 ) ;
#2838=CARTESIAN_POINT ( 'NONE',  ( 2.557341765624996821, -28.40104166700806587, 4.429445870380401828 ) ) ;
#2840=VECTOR ( 'NONE', #2802, 1000.000000000000000 ) ;
#2844=CARTESIAN_POINT ( 'NONE',  ( 6.429395695523604153E-16, -30.00000000000000000, -5.250000000000000000 ) ) ;
#2848=FACE_OUTER_BOUND ( 'NONE', #3562, .T. ) ;
#2849=CARTESIAN_POINT ( 'NONE',  ( -1.406733260263385521, -26.85491455036743247, 5.250000000000006217 ) ) ;
#2855=CARTESIAN_POINT ( 'NONE',  ( 3.616337804771879580E-16, -27.79687500034139802, -5.905927827173866440 ) ) ;
#2857=CARTESIAN_POINT ( 'NONE',  ( 5.250000000000000000, -28.97916666666666430, -3.031088913245534755 ) ) ;
#2859=CARTESIAN_POINT ( 'NONE',  ( -5.114683531250000748, -28.81770833367473017, -2.952963913586935440 ) ) ;
#2860=CARTESIAN_POINT ( 'NONE',  ( -1.084901341431563923E-15, -27.48437500034140157, 5.905927827173866440 ) ) ;
#2865=CARTESIAN_POINT ( 'NONE',  ( 2.557341765624996821, -29.46354166700806232, 4.429445870380401828 ) ) ;
#2869=CARTESIAN_POINT ( 'NONE',  ( 5.114683531249998971, -29.13020833367473372, 2.952963913586936329 ) ) ;
#2870=VERTEX_POINT ( 'NONE', #4817 ) ;
#2875=CARTESIAN_POINT ( 'NONE',  ( -1.406733260263393293, -27.17633545031536713, -5.250000000000000000 ) ) ;
#2879=VECTOR ( 'NONE', #508, 1000.000000000000000 ) ;
#2883=CARTESIAN_POINT ( 'NONE',  ( -2.557341765624999042, -28.77604166700806587, -4.429445870380400052 ) ) ;
#2884=CARTESIAN_POINT ( 'NONE',  ( 5.250000000000000000, -27.53125000068279604, 0.000000000000000000 ) ) ;
#2886=CARTESIAN_POINT ( 'NONE',  ( -1.406733260263387963, -28.95758545099816672, -5.250000000000001776 ) ) ;
#2888=CARTESIAN_POINT ( 'NONE',  ( -1.406733260263382856, -28.20758545099816317, -5.250000000000006217 ) ) ;
#2892=CARTESIAN_POINT ( 'NONE',  ( 2.625000000000000444, -27.20833333333333215, -4.546633369868303021 ) ) ;
#2894=ORIENTED_EDGE ( 'NONE', *, *, #1762, .T. ) ;
#2897=CARTESIAN_POINT ( 'NONE',  ( 2.557341765624996821, -26.90104166700806232, 4.429445870380401828 ) ) ;
#2900=CARTESIAN_POINT ( 'NONE',  ( -1.113604000661152470E-15, -29.56250000000000000, 6.062177826491070398 ) ) ;
#2903=CARTESIAN_POINT ( 'NONE',  ( -2.557341765625002594, -27.75520833367473017, 4.429445870380399164 ) ) ;
#2905=CARTESIAN_POINT ( 'NONE',  ( 2.557341765625000818, -27.63020833367473017, -4.429445870380400052 ) ) ;
#2906=FACE_OUTER_BOUND ( 'NONE', #4988, .T. ) ;
#2908=CARTESIAN_POINT ( 'NONE',  ( 0.000000000000000000, -9.000000000000000000, 0.000000000000000000 ) ) ;
#2912=ORIENTED_EDGE ( 'NONE', *, *, #3174, .T. ) ;
#2915=CARTESIAN_POINT ( 'NONE',  ( -2.557341765625002594, -29.69270833367473017, 4.429445870380399164 ) ) ;
#2918=ORIENTED_EDGE ( 'NONE', *, *, #7856, .F. ) ;
#2922=ORIENTED_EDGE ( 'NONE', *, *, #5548, .F. ) ;
#2923=CARTESIAN_POINT ( 'NONE',  ( 2.300847884672513123E-14, -27.68750000000000000, -5.250000000000000000 ) ) ;
#2926=CARTESIAN_POINT ( 'NONE',  ( -5.114683531249999859, -27.00520833367473017, -2.952963913586935440 ) ) ;
#2938=EDGE_LOOP ( 'NONE', ( #2622, #8965, #3970, #2477 ) ) ;
#2941=ORIENTED_EDGE ( 'NONE', *, *, #7646, .F. ) ;
#2942=CARTESIAN_POINT ( 'NONE',  ( -1.113604000661152470E-15, -28.56249999999999645, 6.062177826491070398 ) ) ;
#2946=CARTESIAN_POINT ( 'NONE',  ( 5.114683531250000748, -28.17187500034139447, 0.000000000000000000 ) ) ;
#2947=CARTESIAN_POINT ( 'NONE',  ( -5.114683531250000748, -28.02604166700806587, 2.952963913586931888 ) ) ;
#2953=CARTESIAN_POINT ( 'NONE',  ( -1.406733260263395735, -27.35491455036742181, 5.250000000000000000 ) ) ;
#2956=ORIENTED_EDGE ( 'NONE', *, *, #2090, .T. ) ;
#2957=CARTESIAN_POINT ( 'NONE',  ( 1.406733260263402174, -28.05133545031536357, 5.249999999999995559 ) ) ;
#2958=CARTESIAN_POINT ( 'NONE',  ( 3.616337804771879580E-16, -28.54687500034139802, -5.905927827173866440 ) ) ;
#2968=CARTESIAN_POINT ( 'NONE',  ( -1.113604000661152470E-15, -29.59375000068279959, 6.062177826491070398 ) ) ;
#2969=CARTESIAN_POINT ( 'NONE',  ( 5.250000000000000000, -29.78125000068279604, 0.000000000000000000 ) ) ;
#2970=CARTESIAN_POINT ( 'NONE',  ( 3.616337804771879580E-16, -29.85937500034139802, -5.905927827173866440 ) ) ;
#2972=CARTESIAN_POINT ( 'NONE',  ( 0.000000000000000000, -9.999999999999998224, 0.000000000000000000 ) ) ;
#2979=CARTESIAN_POINT ( 'NONE',  ( -5.249999999999999112, -27.67708333401612464, -3.031088913245536975 ) ) ;
#2992=CARTESIAN_POINT ( 'NONE',  ( 3.712013335537174572E-16, -28.93749999999999645, -6.062177826491070398 ) ) ;
#2993=CARTESIAN_POINT ( 'NONE',  ( 5.249999999999997335, -29.77083333333332860, 3.031088913245538308 ) ) ;
#2995=CARTESIAN_POINT ( 'NONE',  ( -5.114683531250000748, -27.54687500034139802, -6.263680815196995234E-16 ) ) ;
#2997=CARTESIAN_POINT ( 'NONE',  ( -5.114683531250000748, -27.52604166700806587, 2.952963913586931888 ) ) ;
#3000=CARTESIAN_POINT ( 'NONE',  ( 1.185285273922203525E-14, -28.71875000068279959, -5.250000000000000000 ) ) ;
#3002=CARTESIAN_POINT ( 'NONE',  ( -5.250000000000000000, -29.65625000068279604, -6.429395695523604153E-16 ) ) ;
#3004=EDGE_LOOP ( 'NONE', ( #2783, #9048 ) ) ;
#3007=CARTESIAN_POINT ( 'NONE',  ( -5.114683531250000748, -28.96354166700807298, 2.952963913586931888 ) ) ;
#3008=ORIENTED_EDGE ( 'NONE', *, *, #3394, .T. ) ;
#3009=FACE_OUTER_BOUND ( 'NONE', #6960, .T. ) ;
#3017=PRODUCT_DEFINITION_CONTEXT ( 'detailed design', #5270, 'design' ) ;
#3018=CARTESIAN_POINT ( 'NONE',  ( 5.114683531249998971, -27.38020833367473017, 2.952963913586936329 ) ) ;
#3019=LINE ( 'NONE', #3069, #197 ) ;
#3028=DIRECTION ( 'NONE',  ( 0.000000000000000000, 1.000000000000000000, 0.000000000000000000 ) ) ;
#3031=ORIENTED_EDGE ( 'NONE', *, *, #8536, .F. ) ;
#3033=( BOUNDED_CURVE ( )  B_SPLINE_CURVE ( 2, ( #1588, #3089, #8754, #5065, #891, #6562, #2385, #1494, #7919, #193, #8251, #379, #8294, #3322, #6102, #6005, #4571, #8156, #8932, #330, #3880, #1784, #8799, #3228, #4018, #3828, #8887, #1175, #1884, #3141, #7457, #476, #3272, #4755, #6654, #2581, #6049, #2528, #8844, #5353, #4664, #2481, #8981, #4618, #8202, #2630, #5401, #6702, #425, #6800, #1083, #284, #5449, #3925, #6853, #3971, #4709, #7548, #6153, #1131, #1832, #3184, #1927, #2435, #981, #8106, #5961, #5261, #1734, #5304, #7407, #1030, #6753, #7503, #8519, #7030, #7732, #3454, #3499, #695, #4063, #568, #1223, #7641, #7777, #6939, #8344, #657, #5584, #3367, #3540, #2014, #6322, #9158, #2807, #6283, #7599, #1969, #7684, #2855, #5671, #3412, #5542, #4150, #4798, #1356, #8387, #6902, #6241, #5497, #2717, #5627, #8476, #1308, #6365, #1269, #2101, #526, #9075, #2146, #6985, #4, #4839, #6198, #4924, #4107, #1399, #8428, #4240, #613, #2056, #7071, #4881, #9119, #9026, #2672, #2764, #4195, #1437, #1581, #4329, #3730, #2897, #1629, #2329 ),
 .UNSPECIFIED., .F., .T. ) 
 B_SPLINE_CURVE_WITH_KNOTS ( ( 3, 2, 2, 2, 2, 2, 2, 2, 2, 2, 2, 2, 2, 2, 2, 2, 2, 2, 2, 2, 2, 2, 2, 2, 2, 2, 2, 2, 2, 2, 2, 2, 2, 2, 2, 2, 2, 2, 2, 2, 2, 2, 2, 2, 2, 2, 2, 2, 2, 2, 2, 2, 2, 2, 2, 2, 2, 2, 2, 2, 2, 2, 2, 2, 2, 2, 2, 2, 2, 2, 2, 2, 3 ),
 ( 0.000000000000000000, 0.01388888888888888812, 0.02777777777777777624, 0.04166666666666666435, 0.05555555555555555247, 0.06944444444444444753, 0.08333333333333332871, 0.09722222222222222376, 0.1111111111111111049, 0.1250000000000000000, 0.1388888888888888951, 0.1527777777777777901, 0.1666666666666666574, 0.1805555555555555525, 0.1944444444444444475, 0.2083333333333333426, 0.2222222222222222099, 0.2361111111111111049, 0.2500000000000000000, 0.2638888888888888951, 0.2777777777777777901, 0.2916666666666666852, 0.3055555555555555802, 0.3194444444444444198, 0.3333333333333333148, 0.3472222222222222099, 0.3611111111111111049, 0.3750000000000000000, 0.3888888888888888951, 0.4027777777777777901, 0.4166666666666666852, 0.4305555555555555802, 0.4444444444444444198, 0.4583333333333333148, 0.4722222222222222099, 0.4861111111111111049, 0.5000000000000000000, 0.5138888888888888395, 0.5277777777777777901, 0.5416666666666666297, 0.5555555555555555802, 0.5694444444444444198, 0.5833333333333333703, 0.5972222222222222099, 0.6111111111111111605, 0.6250000000000000000, 0.6388888888888888395, 0.6527777777777777901, 0.6666666666666666297, 0.6805555555555555802, 0.6944444444444444198, 0.7083333333333333703, 0.7222222222222222099, 0.7361111111111111605, 0.7500000000000000000, 0.7638888888888888395, 0.7777777777777777901, 0.7916666666666666297, 0.8055555555555555802, 0.8194444444444444198, 0.8333333333333333703, 0.8472222222222222099, 0.8611111111111111605, 0.8750000000000000000, 0.8888888888888888395, 0.9027777777777777901, 0.9166666666666666297, 0.9305555555555555802, 0.9444444444444444198, 0.9583333333333333703, 0.9722222222222222099, 0.9861111111111111605, 1.000000000000000000 ),
 .UNSPECIFIED. ) 
 CURVE ( )  GEOMETRIC_REPRESENTATION_ITEM ( )  RATIONAL_B_SPLINE_CURVE ( ( 1.000000000000000000, 0.8660254037844387076, 1.000000000000000000, 0.8660254037844387076, 1.000000000000000000, 0.8660254037844387076, 1.000000000000000000, 0.8660254037844387076, 1.000000000000000000, 0.8660254037844387076, 1.000000000000000000, 0.8660254037844387076, 1.000000000000000000, 0.8660254037844387076, 1.000000000000000000, 0.8660254037844387076, 1.000000000000000000, 0.8660254037844387076, 1.000000000000000000, 0.8660254037844387076, 1.000000000000000000, 0.8660254037844387076, 1.000000000000000000, 0.8660254037844387076, 1.000000000000000000, 0.8660254037844387076, 1.000000000000000000, 0.8660254037844387076, 1.000000000000000000, 0.8660254037844387076, 1.000000000000000000, 0.8660254037844387076, 1.000000000000000000, 0.8660254037844387076, 1.000000000000000000, 0.8660254037844387076, 1.000000000000000000, 0.8660254037844387076, 1.000000000000000000, 0.8660254037844387076, 1.000000000000000000, 0.8660254037844387076, 1.000000000000000000, 0.8660254037844387076, 1.000000000000000000, 0.8660254037844387076, 1.000000000000000000, 0.8660254037844387076, 1.000000000000000000, 0.8660254037844387076, 1.000000000000000000, 0.8660254037844387076, 1.000000000000000000, 0.8660254037844387076, 1.000000000000000000, 0.8660254037844387076, 1.000000000000000000, 0.8660254037844387076, 1.000000000000000000, 0.8660254037844387076, 1.000000000000000000, 0.8660254037844387076, 1.000000000000000000, 0.8660254037844387076, 1.000000000000000000, 0.8660254037844387076, 1.000000000000000000, 0.8660254037844387076, 1.000000000000000000, 0.8660254037844387076, 1.000000000000000000, 0.8660254037844387076, 1.000000000000000000, 0.8660254037844387076, 1.000000000000000000, 0.8660254037844387076, 1.000000000000000000, 0.8660254037844387076, 1.000000000000000000, 0.8660254037844387076, 1.000000000000000000, 0.8660254037844387076, 1.000000000000000000, 0.8660254037844387076, 1.000000000000000000, 0.8660254037844387076, 1.000000000000000000, 0.8660254037844387076, 1.000000000000000000, 0.8660254037844387076, 1.000000000000000000, 0.8660254037844387076, 1.000000000000000000, 0.8660254037844387076, 1.000000000000000000, 0.8660254037844387076, 1.000000000000000000, 0.8660254037844387076, 1.000000000000000000, 0.8660254037844387076, 1.000000000000000000, 0.8660254037844387076, 1.000000000000000000, 0.8660254037844387076, 1.000000000000000000, 0.8660254037844387076, 1.000000000000000000, 0.8660254037844387076, 1.000000000000000000, 0.8660254037844387076, 1.000000000000000000, 0.8660254037844387076, 1.000000000000000000, 0.8660254037844387076, 1.000000000000000000, 0.8660254037844387076, 1.000000000000000000, 0.8660254037844387076, 1.000000000000000000, 0.8660254037844387076, 1.000000000000000000, 0.8660254037844387076, 1.000000000000000000, 0.8660254037844387076, 1.000000000000000000, 0.8660254037844387076, 1.000000000000000000, 0.8660254037844387076, 1.000000000000000000, 0.8660254037844387076, 1.000000000000000000, 0.8660254037844387076, 1.000000000000000000, 0.8660254037844387076, 1.000000000000000000, 0.8660254037844387076, 1.000000000000000000, 0.8660254037844387076, 1.000000000000000000, 0.8660254037844387076, 1.000000000000000000, 0.8660254037844387076, 1.000000000000000000, 0.8660254037844387076, 1.000000000000000000 ) ) 
 REPRESENTATION_ITEM ( '' )  );
#3036=VECTOR ( 'NONE', #7187, 1000.000000000000000 ) ;
#3038=ORIENTED_EDGE ( 'NONE', *, *, #1575, .F. ) ;
#3042=CARTESIAN_POINT ( 'NONE',  ( -5.250000000000000000, -28.12499999999999645, -6.429395695523604153E-16 ) ) ;
#3044=CARTESIAN_POINT ( 'NONE',  ( 2.557341765624996821, -28.21354166700806587, 4.429445870380401828 ) ) ;
#3046=CARTESIAN_POINT ( 'NONE',  ( -2.625000000000002220, -29.36458333401613174, 4.546633369868302132 ) ) ;
#3056=CARTESIAN_POINT ( 'NONE',  ( -2.557341765624999042, -28.02604166700806587, -4.429445870380400052 ) ) ;
#3057=VERTEX_POINT ( 'NONE', #2031 ) ;
#3062=CARTESIAN_POINT ( 'NONE',  ( 5.249999999999997335, -27.52083333333332860, 3.031088913245538308 ) ) ;
#3063=ORIENTED_EDGE ( 'NONE', *, *, #905, .F. ) ;
#3065=FACE_OUTER_BOUND ( 'NONE', #1876, .T. ) ;
#3066=CARTESIAN_POINT ( 'NONE',  ( 2.625000000000000444, -28.98958333401613174, -4.546633369868303021 ) ) ;
#3068=CARTESIAN_POINT ( 'NONE',  ( -5.114683531250000748, -27.71354166700806587, 2.952963913586931888 ) ) ;
#3069=CARTESIAN_POINT ( 'NONE',  ( 6.429395695523604153E-16, -30.00000000000000000, -5.250000000000000000 ) ) ;
#3070=DIRECTION ( 'NONE',  ( 0.000000000000000000, 1.000000000000000000, 0.000000000000000000 ) ) ;
#3080=CARTESIAN_POINT ( 'NONE',  ( 2.300847884672513123E-14, -27.43750000000000355, -5.250000000000000000 ) ) ;
#3085=CARTESIAN_POINT ( 'NONE',  ( -5.250000000000000000, -27.89583333333332860, -3.031088913245536531 ) ) ;
#3086=CARTESIAN_POINT ( 'NONE',  ( 3.616337804771879580E-16, -27.85937500034139802, -5.905927827173866440 ) ) ;
#3089=CARTESIAN_POINT ( 'NONE',  ( 5.114683531250000748, -29.83854166700806232, -2.952963913586932776 ) ) ;
#3093=CARTESIAN_POINT ( 'NONE',  ( -1.084901341431563923E-15, -28.23437500034139802, 5.905927827173866440 ) ) ;
#3097=CARTESIAN_POINT ( 'NONE',  ( -5.250000000000000000, -29.37500000000000000, -6.429395695523604153E-16 ) ) ;
#3098=CARTESIAN_POINT ( 'NONE',  ( 3.616337804771879580E-16, -28.79687500034139802, -5.905927827173866440 ) ) ;
#3099=ORIENTED_EDGE ( 'NONE', *, *, #9098, .T. ) ;
#3100=DIRECTION ( 'NONE',  ( 0.000000000000000000, 1.000000000000000000, 0.000000000000000000 ) ) ;
#3101=LINE ( 'NONE', #3841, #41 ) ;
#3103=EDGE_CURVE ( 'NONE', #1439, #3872, #8432, .T. ) ;
#3105=VERTEX_POINT ( 'NONE', #7320 ) ;
#3108=CARTESIAN_POINT ( 'NONE',  ( 5.250000000000000000, -29.28125000068279604, 0.000000000000000000 ) ) ;
#3110=CARTESIAN_POINT ( 'NONE',  ( 5.114683531250000748, -27.60937500034139802, 0.000000000000000000 ) ) ;
#3111=VERTEX_POINT ( 'NONE', #4436 ) ;
#3116=CARTESIAN_POINT ( 'NONE',  ( 5.182341765625000818, -26.82031250051209526, 0.000000000000000000 ) ) ;
#3122=CARTESIAN_POINT ( 'NONE',  ( 1.406733260263405061, -27.69866454968462932, -5.249999999999994671 ) ) ;
#3126=CARTESIAN_POINT ( 'NONE',  ( -2.624999999999998668, -27.41666666666666430, -4.546633369868303021 ) ) ;
#3132=CARTESIAN_POINT ( 'NONE',  ( -5.250000000000000888, -28.10416666666666430, 3.031088913245532979 ) ) ;
#3134=EDGE_CURVE ( 'NONE', #6430, #7910, #1720, .T. ) ;
#3136=ORIENTED_EDGE ( 'NONE', *, *, #2325, .T. ) ;
#3141=CARTESIAN_POINT ( 'NONE',  ( -5.114683531250000748, -29.25520833367473017, -2.952963913586935440 ) ) ;
#3145=CARTESIAN_POINT ( 'NONE',  ( -5.114683531250000748, -28.77604166700806587, 2.952963913586931888 ) ) ;
#3146=ORIENTED_EDGE ( 'NONE', *, *, #5233, .T. ) ;
#3157=CARTESIAN_POINT ( 'NONE',  ( -5.250000000000000888, -29.38541666734946389, 3.031088913245532979 ) ) ;
#3159=ORIENTED_EDGE ( 'NONE', *, *, #5756, .F. ) ;
#3172=VERTEX_POINT ( 'NONE', #6618 ) ;
#3174=EDGE_CURVE ( 'NONE', #7207, #5259, #6830, .T. ) ;
#3176=AXIS2_PLACEMENT_3D ( 'NONE', #833, #4967, #2186 ) ;
#3177=EDGE_LOOP ( 'NONE', ( #3063, #8649, #3733, #1324 ) ) ;
#3178=CARTESIAN_POINT ( 'NONE',  ( 5.249999999999999112, -27.52083333333332860, 3.031088913245538308 ) ) ;
#3179=CARTESIAN_POINT ( 'NONE',  ( -2.557341765625002594, -27.00520833367473017, 4.429445870380399164 ) ) ;
#3184=CARTESIAN_POINT ( 'NONE',  ( 5.114683531250000748, -28.58854166700806587, -2.952963913586932776 ) ) ;
#3187=FACE_OUTER_BOUND ( 'NONE', #1122, .T. ) ;
#3188=CARTESIAN_POINT ( 'NONE',  ( -2.557341765624999042, -28.33854166700806587, -4.429445870380400052 ) ) ;
#3189=CARTESIAN_POINT ( 'NONE',  ( 5.250000000000000000, -27.28125000068279604, 0.000000000000000000 ) ) ;
#3190=AXIS2_PLACEMENT_3D ( 'NONE', #4927, #616, #745 ) ;
#3192=CARTESIAN_POINT ( 'NONE',  ( 2.557341765625000818, -29.88020833367473372, -4.429445870380400052 ) ) ;
#3193=EDGE_LOOP ( 'NONE', ( #9157, #7006 ) ) ;
#3197=CARTESIAN_POINT ( 'NONE',  ( 5.250000000000000000, -30.00000000000000000, 0.000000000000000000 ) ) ;
#3201=CARTESIAN_POINT ( 'NONE',  ( 3.712013335537174572E-16, -27.71875000068279249, -6.062177826491070398 ) ) ;
#3208=DIRECTION ( 'NONE',  ( 0.000000000000000000, 1.000000000000000000, 0.000000000000000000 ) ) ;
#3212=CARTESIAN_POINT ( 'NONE',  ( -2.557341765625002594, -29.44270833367473017, 4.429445870380399164 ) ) ;
#3221=CARTESIAN_POINT ( 'NONE',  ( 5.250000000000000000, -27.72916666666666785, -3.031088913245534755 ) ) ;
#3222=CARTESIAN_POINT ( 'NONE',  ( 1.185285273922203525E-14, -28.71875000068279959, -5.250000000000000000 ) ) ;
#3223=CARTESIAN_POINT ( 'NONE',  ( -5.114683531250000748, -27.04687500034139802, -6.263680815196995234E-16 ) ) ;
#3228=CARTESIAN_POINT ( 'NONE',  ( 5.114683531249998971, -29.38020833367473017, 2.952963913586936329 ) ) ;
#3230=CARTESIAN_POINT ( 'NONE',  ( 2.625000000000000444, -28.48958333401612819, -4.546633369868303021 ) ) ;
#3232=CARTESIAN_POINT ( 'NONE',  ( 5.114683531250000748, -29.17187500034139802, 0.000000000000000000 ) ) ;
#3235=CARTESIAN_POINT ( 'NONE',  ( 2.557341765624996821, -27.65104166700806587, 4.429445870380401828 ) ) ;
#3244=CARTESIAN_POINT ( 'NONE',  ( 0.000000000000000000, -9.999999999999998224, 0.000000000000000000 ) ) ;
#3245=CARTESIAN_POINT ( 'NONE',  ( 2.625000000000000444, -28.23958333401612819, -4.546633369868303021 ) ) ;
#3248=VERTEX_POINT ( 'NONE', #1742 ) ;
#3251=CYLINDRICAL_SURFACE ( 'NONE', #1777, 5.250000000000000000 ) ;
#3255=CARTESIAN_POINT ( 'NONE',  ( 0.000000000000000000, -30.00000000000000000, 5.250000000000000000 ) ) ;
#3264=CARTESIAN_POINT ( 'NONE',  ( 5.250000000000000000, -27.00000000000000000, 0.000000000000000000 ) ) ;
#3268=ORIENTED_EDGE ( 'NONE', *, *, #2410, .F. ) ;
#3269=AXIS2_PLACEMENT_3D ( 'NONE', #490, #3938, #1750 ) ;
#3272=CARTESIAN_POINT ( 'NONE',  ( -2.557341765625002594, -29.19270833367473017, 4.429445870380399164 ) ) ;
#3276=CARTESIAN_POINT ( 'NONE',  ( -2.557341765625002594, -28.75520833367473017, 4.429445870380399164 ) ) ;
#3280=CARTESIAN_POINT ( 'NONE',  ( -2.557341765625002594, -27.44270833367473017, 4.429445870380399164 ) ) ;
#3282=CARTESIAN_POINT ( 'NONE',  ( -1.975475456537005874E-15, -28.31249999999999645, 5.250000000000000000 ) ) ;
#3283=CARTESIAN_POINT ( 'NONE',  ( 5.114683531250000748, -28.42187500034139802, 0.000000000000000000 ) ) ;
#3284=EDGE_LOOP ( 'NONE', ( #5539, #2644, #1775, #2185, #5030, #4984, #2912, #2342, #7253, #669, #7517, #1675, #6620, #2577, #8652, #4081, #8834, #9071, #6380, #9135, #3136, #472, #1799, #3755, #908, #3099, #2894, #3038 ) ) ;
#3292=STYLED_ITEM('',(#9204),#2131);
#3294=CARTESIAN_POINT ( 'NONE',  ( 2.624999999999996891, -27.82291666734946389, 4.546633369868304797 ) ) ;
#3296=ORIENTED_EDGE ( 'NONE', *, *, #3861, .F. ) ;
#3308=( BOUNDED_CURVE ( )  B_SPLINE_CURVE ( 2, ( #6616, #2390, #5121, #6517, #5171, #1692, #4532, #8013, #1740 ),
 .UNSPECIFIED., .F., .T. ) 
 B_SPLINE_CURVE_WITH_KNOTS ( ( 3, 2, 2, 2, 3 ),
 ( 0.4791666666666666852, 0.4861111111111111049, 0.5000000000000000000, 0.5138888888888888395, 0.5208333333333332593 ),
 .UNSPECIFIED. ) 
 CURVE ( )  GEOMETRIC_REPRESENTATION_ITEM ( )  RATIONAL_B_SPLINE_CURVE ( ( 0.9330127018922194093, 0.9330127018922196314, 1.000000000000000000, 0.8660254037844387076, 1.000000000000000000, 0.8660254037844387076, 1.000000000000000000, 0.9330127018922198534, 0.9330127018922192983 ) ) 
 REPRESENTATION_ITEM ( '' )  );
#3312=VERTEX_POINT ( 'NONE', #7463 ) ;
#3313=CARTESIAN_POINT ( 'NONE',  ( 1.406733260263391960, -29.05133545031537068, 5.250000000000000000 ) ) ;
#3322=CARTESIAN_POINT ( 'NONE',  ( 5.114683531250000748, -29.58854166700806232, -2.952963913586932776 ) ) ;
#3324=CYLINDRICAL_SURFACE ( 'NONE', #1239, 5.250000000000000000 ) ;
#3325=CARTESIAN_POINT ( 'NONE',  ( 5.114683531250000748, -27.92187500034139802, 0.000000000000000000 ) ) ;
#3328=CARTESIAN_POINT ( 'NONE',  ( 5.114683531249999859, -27.08854166700806232, -2.952963913586932776 ) ) ;
#3329=CARTESIAN_POINT ( 'NONE',  ( 2.033577675846918216E-14, -27.06250000000000355, 5.250000000000000888 ) ) ;
#3330=CARTESIAN_POINT ( 'NONE',  ( -5.114683531250000748, -29.29687500034139802, -6.263680815196995234E-16 ) ) ;
#3331=EDGE_CURVE ( 'NONE', #2547, #3693, #1127, .T. ) ;
#3335=CARTESIAN_POINT ( 'NONE',  ( -5.250000000000000000, -29.15625000068279604, -6.429395695523604153E-16 ) ) ;
#3336=CIRCLE ( 'NONE', #7185, 4.250000000000000000 ) ;
#3341=VERTEX_POINT ( 'NONE', #6708 ) ;
#3343=CARTESIAN_POINT ( 'NONE',  ( -2.625000000000002220, -28.61458333401612819, 4.546633369868302132 ) ) ;
#3348=CARTESIAN_POINT ( 'NONE',  ( 1.406733260263394625, -29.72991455036742536, -5.250000000000000000 ) ) ;
#3349=EDGE_CURVE ( 'NONE', #5259, #627, #5870, .T. ) ;
#3361=EDGE_LOOP ( 'NONE', ( #541, #7887, #9182, #3588 ) ) ;
#3363=DIRECTION ( 'NONE',  ( 0.000000000000000000, 1.000000000000000000, 0.000000000000000000 ) ) ;
#3365=VERTEX_POINT ( 'NONE', #5406 ) ;
#3367=CARTESIAN_POINT ( 'NONE',  ( -5.114683531250000748, -28.00520833367473017, -2.952963913586935440 ) ) ;
#3370=CARTESIAN_POINT ( 'NONE',  ( 5.114683531250000748, -27.67187500034139802, 0.000000000000000000 ) ) ;
#3372=CARTESIAN_POINT ( 'NONE',  ( -2.557341765625002594, -29.75520833367473017, 4.429445870380399164 ) ) ;
#3373=CARTESIAN_POINT ( 'NONE',  ( 2.624999999999996891, -27.04166666666666430, 4.546633369868304797 ) ) ;
#3374=CARTESIAN_POINT ( 'NONE',  ( 2.557341765625000818, -28.38020833367473017, -4.429445870380400052 ) ) ;
#3384=DIRECTION ( 'NONE',  ( 0.000000000000000000, 1.000000000000000000, 0.000000000000000000 ) ) ;
#3385=CARTESIAN_POINT ( 'NONE',  ( -2.625000000000002220, -28.11458333401612819, 4.546633369868302132 ) ) ;
#3387=( BOUNDED_CURVE ( )  B_SPLINE_CURVE ( 2, ( #8243, #3313, #4701, #3407, #9068, #4188, #3492, #7021, #1350 ),
 .UNSPECIFIED., .F., .T. ) 
 B_SPLINE_CURVE_WITH_KNOTS ( ( 3, 2, 2, 2, 3 ),
 ( 0.3125000000000000000, 0.3194444444444444198, 0.3333333333333333148, 0.3472222222222222099, 0.3541666666666666297 ),
 .UNSPECIFIED. ) 
 CURVE ( )  GEOMETRIC_REPRESENTATION_ITEM ( )  RATIONAL_B_SPLINE_CURVE ( ( 0.9330127018922194093, 0.9330127018922194093, 1.000000000000000000, 0.8660254037844387076, 1.000000000000000000, 0.8660254037844387076, 1.000000000000000000, 0.9330127018922196314, 0.9330127018922194093 ) ) 
 REPRESENTATION_ITEM ( '' )  );
#3393=DIRECTION ( 'NONE',  ( 0.000000000000000000, 1.000000000000000000, 0.000000000000000000 ) ) ;
#3394=EDGE_CURVE ( 'NONE', #2074, #4147, #1526, .T. ) ;
#3395=DIRECTION ( 'NONE',  ( 0.000000000000000000, -0.000000000000000000, 1.000000000000000000 ) ) ;
#3398=CARTESIAN_POINT ( 'NONE',  ( 5.114683531250000748, -29.60937500034139802, 0.000000000000000000 ) ) ;
#3399=CARTESIAN_POINT ( 'NONE',  ( 2.624999999999996891, -27.57291666734946389, 4.546633369868304797 ) ) ;
#3400=PRODUCT_CONTEXT ( 'NONE', #525, 'mechanical' ) ;
#3407=CARTESIAN_POINT ( 'NONE',  ( 5.249999999999997335, -29.02083333333332860, 3.031088913245538308 ) ) ;
#3408=FACE_OUTER_BOUND ( 'NONE', #378, .T. ) ;
#3412=CARTESIAN_POINT ( 'NONE',  ( -5.114683531250000748, -27.75520833367473017, -2.952963913586935440 ) ) ;
#3415=CARTESIAN_POINT ( 'NONE',  ( 2.557341765624996821, -27.96354166700806587, 4.429445870380401828 ) ) ;
#3416=CARTESIAN_POINT ( 'NONE',  ( 2.300847884672513123E-14, -27.21875000068279959, -5.250000000000000000 ) ) ;
#3417=EDGE_CURVE ( 'NONE', #5951, #7705, #1393, .T. ) ;
#3418=CARTESIAN_POINT ( 'NONE',  ( -1.084901341431563726E-15, -28.73437500034139802, 5.905927827173866440 ) ) ;
#3421=CARTESIAN_POINT ( 'NONE',  ( 5.114683531249999859, -29.40104166700806232, -2.952963913586932776 ) ) ;
#3425=CARTESIAN_POINT ( 'NONE',  ( 1.406733260263391960, -28.83258545099816672, 5.250000000000000000 ) ) ;
#3432=CARTESIAN_POINT ( 'NONE',  ( 5.114683531249999859, -29.83854166700806587, -2.952963913586932776 ) ) ;
#3443=CARTESIAN_POINT ( 'NONE',  ( -1.084901341431563923E-15, -28.67187500034139802, 5.905927827173866440 ) ) ;
#3446=EDGE_CURVE ( 'NONE', #7910, #4820, #8491, .T. ) ;
#3450=DIRECTION ( 'NONE',  ( 0.000000000000000000, 1.000000000000000000, 0.000000000000000000 ) ) ;
#3454=CARTESIAN_POINT ( 'NONE',  ( -5.114683531250000748, -28.25520833367473017, -2.952963913586935440 ) ) ;
#3456=CARTESIAN_POINT ( 'NONE',  ( -1.084901341431563923E-15, -27.23437500034139802, 5.905927827173866440 ) ) ;
#3457=CARTESIAN_POINT ( 'NONE',  ( 0.000000000000000000, -30.00000000000000000, 5.250000000000000000 ) ) ;
#3458=CARTESIAN_POINT ( 'NONE',  ( -2.557341765625002594, -29.25520833367473017, 4.429445870380399164 ) ) ;
#3461=CARTESIAN_POINT ( 'NONE',  ( 3.616337804771879580E-16, -29.60937500034139447, -5.905927827173866440 ) ) ;
#3462=CARTESIAN_POINT ( 'NONE',  ( -1.406733260263393293, -28.45758545099816672, -5.250000000000000000 ) ) ;
#3465=CARTESIAN_POINT ( 'NONE',  ( 1.406733260263391960, -29.58258545099816317, 5.250000000000000000 ) ) ;
#3472=CARTESIAN_POINT ( 'NONE',  ( -5.250000000000000888, -26.88541666734946389, 3.031088913245532979 ) ) ;
#3478=CARTESIAN_POINT ( 'NONE',  ( -5.249999999999999112, -27.14583333333332860, -3.031088913245536975 ) ) ;
#3484=CARTESIAN_POINT ( 'NONE',  ( -1.084901341431563923E-15, -29.17187500034139802, 5.905927827173866440 ) ) ;
#3485=DIRECTION ( 'NONE',  ( -0.000000000000000000, -1.000000000000000000, -0.000000000000000000 ) ) ;
#3489=CARTESIAN_POINT ( 'NONE',  ( -2.625000000000002220, -28.11458333401612819, 4.546633369868302132 ) ) ;
#3492=CARTESIAN_POINT ( 'NONE',  ( 2.625000000000000444, -28.95833333333333215, -4.546633369868303021 ) ) ;
#3497=EDGE_CURVE ( 'NONE', #3872, #2716, #1416, .T. ) ;
#3499=CARTESIAN_POINT ( 'NONE',  ( -5.114683531250000748, -28.23437500034139447, -6.263680815196995234E-16 ) ) ;
#3501=CARTESIAN_POINT ( 'NONE',  ( -2.557341765624999042, -27.33854166700806587, -4.429445870380400052 ) ) ;
#3503=EDGE_CURVE ( 'NONE', #4350, #4963, #7874, .T. ) ;
#3504=CARTESIAN_POINT ( 'NONE',  ( 5.114683531250000748, -29.40104166700806232, -2.952963913586932776 ) ) ;
#3506=CARTESIAN_POINT ( 'NONE',  ( -2.557341765624999042, -27.83854166700806587, -4.429445870380400052 ) ) ;
#3511=CARTESIAN_POINT ( 'NONE',  ( 0.000000000000000000, -9.999999999999998224, 4.250000000000000000 ) ) ;
#3516=CARTESIAN_POINT ( 'NONE',  ( 2.624999999999996891, -27.32291666734946389, 4.546633369868304797 ) ) ;
#3517=ORIENTED_EDGE ( 'NONE', *, *, #7310, .T. ) ;
#3520=CARTESIAN_POINT ( 'NONE',  ( -2.625000000000002220, -27.08333333333333570, 4.546633369868302132 ) ) ;
#3528=CARTESIAN_POINT ( 'NONE',  ( -2.557341765625002594, -28.69270833367473017, 4.429445870380399164 ) ) ;
#3537=ORIENTED_EDGE ( 'NONE', *, *, #6341, .T. ) ;
#3540=CARTESIAN_POINT ( 'NONE',  ( -5.114683531250000748, -27.98437500034139802, -6.263680815196995234E-16 ) ) ;
#3542=CARTESIAN_POINT ( 'NONE',  ( 5.250000000000000000, -29.25000000000000000, 0.000000000000000000 ) ) ;
#3544=( BOUNDED_CURVE ( )  B_SPLINE_CURVE ( 2, ( #6657, #5119, #1690, #1642, #2388, #4481, #6614, #8011, #2338 ),
 .UNSPECIFIED., .F., .T. ) 
 B_SPLINE_CURVE_WITH_KNOTS ( ( 3, 2, 2, 2, 3 ),
 ( 0.3958333333333333703, 0.4027777777777777901, 0.4166666666666666852, 0.4305555555555555802, 0.4375000000000000000 ),
 .UNSPECIFIED. ) 
 CURVE ( )  GEOMETRIC_REPRESENTATION_ITEM ( )  RATIONAL_B_SPLINE_CURVE ( ( 0.9330127018922194093, 0.9330127018922196314, 1.000000000000000000, 0.8660254037844387076, 1.000000000000000000, 0.8660254037844387076, 1.000000000000000000, 0.9330127018922194093, 0.9330127018922194093 ) ) 
 REPRESENTATION_ITEM ( '' )  );
#3545=CARTESIAN_POINT ( 'NONE',  ( -1.084901341431563726E-15, -28.98437500034139802, 5.905927827173866440 ) ) ;
#3546=( NAMED_UNIT ( * ) SI_UNIT ( $, .STERADIAN. ) SOLID_ANGLE_UNIT ( ) );
#3549=CARTESIAN_POINT ( 'NONE',  ( -5.114683531249999859, -27.06770833367473017, -2.952963913586935440 ) ) ;
#3553=EDGE_CURVE ( 'NONE', #566, #849, #1179, .T. ) ;
#3558=VECTOR ( 'NONE', #3949, 1000.000000000000000 ) ;
#3560=CARTESIAN_POINT ( 'NONE',  ( -2.557341765624999042, -29.77604166700806232, -4.429445870380400052 ) ) ;
#3562=EDGE_LOOP ( 'NONE', ( #4564, #547 ) ) ;
#3566=CARTESIAN_POINT ( 'NONE',  ( 7.041719095097280880E-16, -9.999999999999998224, -5.750000000000000000 ) ) ;
#3569=DIRECTION ( 'NONE',  ( 0.000000000000000000, 1.000000000000000000, 0.000000000000000000 ) ) ;
#3570=CARTESIAN_POINT ( 'NONE',  ( 2.033577675846918216E-14, -28.06249999999999645, 5.250000000000000888 ) ) ;
#3572=CARTESIAN_POINT ( 'NONE',  ( -5.114683531249999859, -28.25520833367473017, -2.952963913586935440 ) ) ;
#3575=CARTESIAN_POINT ( 'NONE',  ( 1.406733260263400176, -28.97991455036743247, -5.249999999999997335 ) ) ;
#3582=CARTESIAN_POINT ( 'NONE',  ( -5.250000000000000888, -26.88541666734946389, 3.031088913245533423 ) ) ;
#3585=VERTEX_POINT ( 'NONE', #7158 ) ;
#3588=ORIENTED_EDGE ( 'NONE', *, *, #4748, .F. ) ;
#3589=CARTESIAN_POINT ( 'NONE',  ( 2.625000000000000444, -28.95833333333333215, -4.546633369868303021 ) ) ;
#3591=ADVANCED_FACE ( 'NONE', ( #3629 ), #6451, .T. ) ;
#3592=CARTESIAN_POINT ( 'NONE',  ( -5.114683531250000748, -27.79687500034139802, -6.263680815196995234E-16 ) ) ;
#3593=CARTESIAN_POINT ( 'NONE',  ( 2.557341765624996821, -27.96354166700806587, 4.429445870380401828 ) ) ;
#3594=DIRECTION ( 'NONE',  ( 0.000000000000000000, 1.000000000000000000, 0.000000000000000000 ) ) ;
#3598=CARTESIAN_POINT ( 'NONE',  ( 0.000000000000000000, -9.999999999999998224, 5.250000000000000000 ) ) ;
#3599=CARTESIAN_POINT ( 'NONE',  ( -5.114683531250000748, -29.52604166700806232, 2.952963913586931888 ) ) ;
#3604=CARTESIAN_POINT ( 'NONE',  ( 5.250000000000000000, -27.28125000068279604, 0.000000000000000000 ) ) ;
#3610=CARTESIAN_POINT ( 'NONE',  ( 2.300847884672513123E-14, -27.68750000000000355, -5.250000000000000000 ) ) ;
#3613=CARTESIAN_POINT ( 'NONE',  ( -5.250000000000000888, -27.60416666666666430, 3.031088913245533423 ) ) ;
#3614=VECTOR ( 'NONE', #8286, 1000.000000000000000 ) ;
#3616=CARTESIAN_POINT ( 'NONE',  ( 2.033577675846918216E-14, -27.84375000068279959, 5.250000000000000888 ) ) ;
#3618=CARTESIAN_POINT ( 'NONE',  ( -2.557341765625002594, -27.19270833367473017, 4.429445870380399164 ) ) ;
#3619=DIRECTION ( 'NONE',  ( 0.000000000000000000, 1.000000000000000000, 0.000000000000000000 ) ) ;
#3627=VECTOR ( 'NONE', #7104, 1000.000000000000114 ) ;
#3628=CARTESIAN_POINT ( 'NONE',  ( 0.000000000000000000, -9.999999999999998224, 0.000000000000000000 ) ) ;
#3629=FACE_OUTER_BOUND ( 'NONE', #2446, .T. ) ;
#3637=CARTESIAN_POINT ( 'NONE',  ( -5.250000000000000000, -28.62499999999999645, -6.429395695523604153E-16 ) ) ;
#3638=DIRECTION ( 'NONE',  ( 0.000000000000000000, 1.000000000000000000, 0.000000000000000000 ) ) ;
#3639=CARTESIAN_POINT ( 'NONE',  ( 5.114683531250000748, -27.40104166700806587, -2.952963913586932776 ) ) ;
#3640=CARTESIAN_POINT ( 'NONE',  ( -5.114683531249999859, -28.06770833367473017, -2.952963913586935440 ) ) ;
#3647=ORIENTED_EDGE ( 'NONE', *, *, #7606, .F. ) ;
#3648=CARTESIAN_POINT ( 'NONE',  ( -1.406733260263390628, -28.60491455036742892, 5.250000000000001776 ) ) ;
#3649=CARTESIAN_POINT ( 'NONE',  ( -1.084901341431563923E-15, -28.67187500034139802, 5.905927827173866440 ) ) ;
#3657=CARTESIAN_POINT ( 'NONE',  ( -2.624999999999998668, -29.19791666734946389, -4.546633369868303021 ) ) ;
#3661=CARTESIAN_POINT ( 'NONE',  ( 5.114683531249999859, -29.90104166700806232, -2.952963913586932776 ) ) ;
#3665=EDGE_CURVE ( 'NONE', #8002, #2547, #2126, .T. ) ;
#3666=DIRECTION ( 'NONE',  ( 0.000000000000000000, 0.000000000000000000, 1.000000000000000000 ) ) ;
#3670=DIRECTION ( 'NONE',  ( -0.000000000000000000, -1.000000000000000000, -0.000000000000000000 ) ) ;
#3672=ORIENTED_EDGE ( 'NONE', *, *, #7646, .T. ) ;
#3674=( BOUNDED_CURVE ( )  B_SPLINE_CURVE ( 2, ( #2923, #4177, #1513, #5039, #2213, #3613, #4949, #2081, #5740 ),
 .UNSPECIFIED., .F., .T. ) 
 B_SPLINE_CURVE_WITH_KNOTS ( ( 3, 2, 2, 2, 3 ),
 ( 0.7708333333333332593, 0.7777777777777777901, 0.7916666666666666297, 0.8055555555555555802, 0.8125000000000000000 ),
 .UNSPECIFIED. ) 
 CURVE ( )  GEOMETRIC_REPRESENTATION_ITEM ( )  RATIONAL_B_SPLINE_CURVE ( ( 0.9330127018922192983, 0.9330127018922187432, 1.000000000000000000, 0.8660254037844387076, 1.000000000000000000, 0.8660254037844387076, 1.000000000000000000, 0.9330127018922194093, 0.9330127018922194093 ) ) 
 REPRESENTATION_ITEM ( '' )  );
#3677=ORIENTED_EDGE ( 'NONE', *, *, #4836, .F. ) ;
#3680=ORIENTED_EDGE ( 'NONE', *, *, #3665, .F. ) ;
#3681=CARTESIAN_POINT ( 'NONE',  ( 5.249999999999999112, -29.27083333333333215, 3.031088913245538308 ) ) ;
#3682=CARTESIAN_POINT ( 'NONE',  ( -1.975475456537005874E-15, -29.81249999999999645, 5.250000000000000000 ) ) ;
#3683=CARTESIAN_POINT ( 'NONE',  ( 5.114683531250000748, -27.92187500034139802, 0.000000000000000000 ) ) ;
#3684=CARTESIAN_POINT ( 'NONE',  ( 5.114683531249999859, -27.40104166700806587, -2.952963913586932776 ) ) ;
#3688=DIRECTION ( 'NONE',  ( 0.000000000000000000, 0.000000000000000000, 1.000000000000000000 ) ) ;
#3689=DIRECTION ( 'NONE',  ( 0.000000000000000000, 1.000000000000000000, 0.000000000000000000 ) ) ;
#3691=CARTESIAN_POINT ( 'NONE',  ( 5.249999999999997335, -27.30208333401612819, 3.031088913245538308 ) ) ;
#3693=VERTEX_POINT ( 'NONE', #6780 ) ;
#3695=CARTESIAN_POINT ( 'NONE',  ( 1.406733260263394625, -27.94866454968462222, -5.250000000000000000 ) ) ;
#3696=CARTESIAN_POINT ( 'NONE',  ( -2.557341765624999042, -28.77604166700806587, -4.429445870380400052 ) ) ;
#3700=CARTESIAN_POINT ( 'NONE',  ( 6.429395695523604153E-16, -30.00000000000000000, -5.250000000000000000 ) ) ;
#3703=CARTESIAN_POINT ( 'NONE',  ( 6.972266317189433020E-16, -29.21875000068279249, -5.249999999999999112 ) ) ;
#3705=VERTEX_POINT ( 'NONE', #406 ) ;
#3707=CARTESIAN_POINT ( 'NONE',  ( 5.250000000000000000, -29.78125000068279604, 0.000000000000000000 ) ) ;
#3709=AXIS2_PLACEMENT_3D ( 'NONE', #7611, #346, #4077 ) ;
#3710=CARTESIAN_POINT ( 'NONE',  ( -2.557341765624999042, -27.27604166700806587, -4.429445870380400052 ) ) ;
#3728=CARTESIAN_POINT ( 'NONE',  ( 0.000000000000000000, -30.00000000000000000, 0.000000000000000000 ) ) ;
#3729=ORIENTED_EDGE ( 'NONE', *, *, #7817, .T. ) ;
#3730=CARTESIAN_POINT ( 'NONE',  ( -1.084901341431563726E-15, -26.92187500034139802, 5.905927827173866440 ) ) ;
#3733=ORIENTED_EDGE ( 'NONE', *, *, #2410, .T. ) ;
#3734=CARTESIAN_POINT ( 'NONE',  ( -2.625000000000002220, -29.08333333333333215, 4.546633369868302132 ) ) ;
#3736=CARTESIAN_POINT ( 'NONE',  ( -1.084901341431563726E-15, -27.73437500034139802, 5.905927827173866440 ) ) ;
#3738=AXIS2_PLACEMENT_3D ( 'NONE', #4920, #5754, #7769 ) ;
#3739=CARTESIAN_POINT ( 'NONE',  ( -5.249999999999999112, -29.42708333401613174, -3.031088913245536975 ) ) ;
#3747=ORIENTED_EDGE ( 'NONE', *, *, #4815, .T. ) ;
#3748=CARTESIAN_POINT ( 'NONE',  ( 5.250000000000000000, -27.03125000068279604, 0.000000000000000000 ) ) ;
#3749=CARTESIAN_POINT ( 'NONE',  ( -2.557341765624999042, -29.02604166700806587, -4.429445870380400052 ) ) ;
#3750=ORIENTED_EDGE ( 'NONE', *, *, #609, .F. ) ;
#3754=CARTESIAN_POINT ( 'NONE',  ( 1.406733260263405061, -27.44866454968462932, -5.249999999999994671 ) ) ;
#3755=ORIENTED_EDGE ( 'NONE', *, *, #2044, .T. ) ;
#3757=CARTESIAN_POINT ( 'NONE',  ( 3.712013335537174572E-16, -29.21875000068279249, -6.062177826491070398 ) ) ;
#3759=CARTESIAN_POINT ( 'NONE',  ( -5.114683531250000748, -29.77604166700806232, 2.952963913586931888 ) ) ;
#3763=UNCERTAINTY_MEASURE_WITH_UNIT (LENGTH_MEASURE( 1.000000000000000082E-05 ), #145, 'distance_accuracy_value', 'NONE');
#3766=AXIS2_PLACEMENT_3D ( 'NONE', #6927, #1112, #5380 ) ;
#3781=CARTESIAN_POINT ( 'NONE',  ( 5.249999999999999112, -27.27083333333332860, 3.031088913245538308 ) ) ;
#3783=CARTESIAN_POINT ( 'NONE',  ( 5.114683531249998971, -27.69270833367473017, 2.952963913586936329 ) ) ;
#3785=CARTESIAN_POINT ( 'NONE',  ( -1.084901341431563923E-15, -26.98437500034139802, 5.905927827173866440 ) ) ;
#3786=DIRECTION ( 'NONE',  ( 0.000000000000000000, 1.000000000000000000, 0.000000000000000000 ) ) ;
#3791=CARTESIAN_POINT ( 'NONE',  ( -5.114683531249999859, -28.31770833367473372, -2.952963913586935440 ) ) ;
#3795=CARTESIAN_POINT ( 'NONE',  ( 5.114683531250000748, -28.60937500034139802, 0.000000000000000000 ) ) ;
#3802=VERTEX_POINT ( 'NONE', #2969 ) ;
#3803=FACE_OUTER_BOUND ( 'NONE', #7304, .T. ) ;
#3805=CARTESIAN_POINT ( 'NONE',  ( 5.114683531249998971, -27.88020833367473017, 2.952963913586936329 ) ) ;
#3807=DIRECTION ( 'NONE',  ( 0.000000000000000000, 0.000000000000000000, 1.000000000000000000 ) ) ;
#3809=DIRECTION ( 'NONE',  ( 0.8660254037844402619, -0.4999999999999970579, 0.000000000000000000 ) ) ;
#3812=CARTESIAN_POINT ( 'NONE',  ( 3.367778697655221012E-16, -9.999999999999998224, -2.750000000000000000 ) ) ;
#3824=CARTESIAN_POINT ( 'NONE',  ( 5.249999999999999112, -28.02083333333333215, 3.031088913245538308 ) ) ;
#3828=CARTESIAN_POINT ( 'NONE',  ( 5.114683531250000748, -29.33854166700806232, -2.952963913586932776 ) ) ;
#3830=LINE ( 'NONE', #2387, #2829 ) ;
#3831=CARTESIAN_POINT ( 'NONE',  ( 2.300847884672513123E-14, -27.46875000068279604, -5.250000000000000000 ) ) ;
#3832=CARTESIAN_POINT ( 'NONE',  ( -1.084901341431563923E-15, -29.23437500034139802, 5.905927827173866440 ) ) ;
#3835=CARTESIAN_POINT ( 'NONE',  ( 6.972266317189433020E-16, -26.96875000068279249, -5.250000000000000000 ) ) ;
#3836=CARTESIAN_POINT ( 'NONE',  ( -2.557341765625002594, -28.19270833367473017, 4.429445870380399164 ) ) ;
#3838=ORIENTED_EDGE ( 'NONE', *, *, #5661, .F. ) ;
#3841=CARTESIAN_POINT ( 'NONE',  ( 5.204748896376250699E-16, -30.00000000000000000, -4.250000000000000000 ) ) ;
#3846=( BOUNDED_CURVE ( )  B_SPLINE_CURVE ( 2, ( #2348, #5178, #853, #8581, #8069 ),
 .UNSPECIFIED., .F., .F. ) 
 B_SPLINE_CURVE_WITH_KNOTS ( ( 3, 2, 3 ),
 ( 0.9791666666666667407, 0.9861111111111111605, 1.000000000000000000 ),
 .UNSPECIFIED. ) 
 CURVE ( )  GEOMETRIC_REPRESENTATION_ITEM ( )  RATIONAL_B_SPLINE_CURVE ( ( 0.9330127018922192983, 0.9330127018922198534, 1.000000000000000000, 0.8660254037844387076, 1.000000000000000000 ) ) 
 REPRESENTATION_ITEM ( '' )  );
#3848=CARTESIAN_POINT ( 'NONE',  ( -2.624999999999998668, -29.69791666734946034, -4.546633369868303021 ) ) ;
#3851=CARTESIAN_POINT ( 'NONE',  ( -5.114683531249999859, -29.56770833367473017, -2.952963913586935440 ) ) ;
#3853=VECTOR ( 'NONE', #1936, 1000.000000000000000 ) ;
#3861=EDGE_CURVE ( 'NONE', #3693, #566, #5272, .T. ) ;
#3862=CARTESIAN_POINT ( 'NONE',  ( 0.000000000000000000, 75.00000000000000000, 4.250000000000000000 ) ) ;
#3863=DIRECTION ( 'NONE',  ( 0.000000000000000000, 0.000000000000000000, 1.000000000000000000 ) ) ;
#3872=VERTEX_POINT ( 'NONE', #8544 ) ;
#3873=CARTESIAN_POINT ( 'NONE',  ( 2.624999999999996891, -27.54166666666666430, 4.546633369868304797 ) ) ;
#3876=EDGE_LOOP ( 'NONE', ( #6690, #4126, #7029, #3268 ) ) ;
#3880=CARTESIAN_POINT ( 'NONE',  ( -2.557341765625002594, -29.44270833367473017, 4.429445870380399164 ) ) ;
#3884=CARTESIAN_POINT ( 'NONE',  ( 5.114683531249999859, -28.90104166700806942, -2.952963913586932776 ) ) ;
#3887=CARTESIAN_POINT ( 'NONE',  ( 1.406733260263400176, -29.19866454968462932, -5.249999999999997335 ) ) ;
#3889=CARTESIAN_POINT ( 'NONE',  ( -2.557341765625002594, -27.69270833367473017, 4.429445870380399164 ) ) ;
#3898=CARTESIAN_POINT ( 'NONE',  ( -5.250000000000000888, -28.63541666734946389, 3.031088913245532979 ) ) ;
#3904=( BOUNDED_CURVE ( )  B_SPLINE_CURVE ( 2, ( #6877, #9005, #505, #3348, #5473 ),
 .UNSPECIFIED., .F., .F. ) 
 B_SPLINE_CURVE_WITH_KNOTS ( ( 3, 2, 3 ),
 ( 0.000000000000000000, 0.01388888888888888812, 0.02083333333333333218 ),
 .UNSPECIFIED. ) 
 CURVE ( )  GEOMETRIC_REPRESENTATION_ITEM ( )  RATIONAL_B_SPLINE_CURVE ( ( 1.000000000000000000, 0.8660254037844387076, 1.000000000000000000, 0.9330127018922194093, 0.9330127018922194093 ) ) 
 REPRESENTATION_ITEM ( '' )  );
#3906=FACE_OUTER_BOUND ( 'NONE', #19, .T. ) ;
#3909=CARTESIAN_POINT ( 'NONE',  ( -2.557341765624999042, -29.52604166700806232, -4.429445870380400052 ) ) ;
#3913=AXIS2_PLACEMENT_3D ( 'NONE', #640, #3485, #8326 ) ;
#3918=CARTESIAN_POINT ( 'NONE',  ( -5.250000000000000000, -27.64583333333333215, -3.031088913245536531 ) ) ;
#3923=CARTESIAN_POINT ( 'NONE',  ( -2.624999999999998668, -29.44791666734946034, -4.546633369868303021 ) ) ;
#3924=ORIENTED_EDGE ( 'NONE', *, *, #4012, .F. ) ;
#3925=CARTESIAN_POINT ( 'NONE',  ( -5.114683531250000748, -28.75520833367473017, -2.952963913586935440 ) ) ;
#3929=CARTESIAN_POINT ( 'NONE',  ( 2.557341765624996821, -28.96354166700806587, 4.429445870380401828 ) ) ;
#3933=CARTESIAN_POINT ( 'NONE',  ( -2.557341765624999042, -27.52604166700806587, -4.429445870380400052 ) ) ;
#3934=ORIENTED_EDGE ( 'NONE', *, *, #1538, .F. ) ;
#3938=DIRECTION ( 'NONE',  ( 0.000000000000000000, 1.000000000000000000, 0.000000000000000000 ) ) ;
#3941=ORIENTED_EDGE ( 'NONE', *, *, #7926, .F. ) ;
#3943=CARTESIAN_POINT ( 'NONE',  ( -5.250000000000000000, -27.42708333401613174, -3.031088913245536531 ) ) ;
#3949=DIRECTION ( 'NONE',  ( 0.000000000000000000, 1.000000000000000000, 0.000000000000000000 ) ) ;
#3951=CARTESIAN_POINT ( 'NONE',  ( -5.250000000000000000, -28.87499999999999645, -6.429395695523604153E-16 ) ) ;
#3952=CARTESIAN_POINT ( 'NONE',  ( 6.429395695523604153E-16, -30.00000000000000000, -5.250000000000000000 ) ) ;
#3954=CARTESIAN_POINT ( 'NONE',  ( 5.114683531250000748, -29.85937500034139802, 0.000000000000000000 ) ) ;
#3955=CARTESIAN_POINT ( 'NONE',  ( 2.300847884672513123E-14, -27.68750000000000000, -5.250000000000000000 ) ) ;
#3959=EDGE_CURVE ( 'NONE', #2168, #8645, #5723, .T. ) ;
#3966=CARTESIAN_POINT ( 'NONE',  ( 2.557341765625000818, -27.13020833367473017, -4.429445870380400052 ) ) ;
#3970=ORIENTED_EDGE ( 'NONE', *, *, #7418, .F. ) ;
#3971=CARTESIAN_POINT ( 'NONE',  ( -5.114683531250001636, -28.71354166700806587, 2.952963913586931444 ) ) ;
#3973=CARTESIAN_POINT ( 'NONE',  ( 5.250000000000000000, -28.53125000068279604, 0.000000000000000000 ) ) ;
#3975=CARTESIAN_POINT ( 'NONE',  ( 2.557341765625000818, -29.13020833367473017, -4.429445870380400052 ) ) ;
#3978=CARTESIAN_POINT ( 'NONE',  ( 2.557341765624996821, -27.40104166700806587, 4.429445870380401828 ) ) ;
#3980=( BOUNDED_CURVE ( )  B_SPLINE_CURVE ( 2, ( #815, #1051, #1195, #1898, #7616, #6820, #497, #8313, #8997 ),
 .UNSPECIFIED., .F., .T. ) 
 B_SPLINE_CURVE_WITH_KNOTS ( ( 3, 2, 2, 2, 3 ),
 ( 0.1458333333333333426, 0.1527777777777777901, 0.1666666666666666574, 0.1805555555555555525, 0.1875000000000000000 ),
 .UNSPECIFIED. ) 
 CURVE ( )  GEOMETRIC_REPRESENTATION_ITEM ( )  RATIONAL_B_SPLINE_CURVE ( ( 0.9330127018922194093, 0.9330127018922194093, 1.000000000000000000, 0.8660254037844387076, 1.000000000000000000, 0.8660254037844387076, 1.000000000000000000, 0.9330127018922194093, 0.9330127018922194093 ) ) 
 REPRESENTATION_ITEM ( '' )  );
#3981=( GEOMETRIC_REPRESENTATION_CONTEXT ( 3 ) GLOBAL_UNCERTAINTY_ASSIGNED_CONTEXT ( ( #8685 ) ) GLOBAL_UNIT_ASSIGNED_CONTEXT ( ( #1080, #1684, #7454 ) ) REPRESENTATION_CONTEXT ( 'NONE', 'WORKASPACE' ) );
#3982=DIRECTION ( 'NONE',  ( 0.000000000000000000, 0.000000000000000000, 1.000000000000000000 ) ) ;
#3991=CARTESIAN_POINT ( 'NONE',  ( -5.250000000000000888, -28.38541666734946034, 3.031088913245532979 ) ) ;
#3993=ORIENTED_EDGE ( 'NONE', *, *, #4097, .F. ) ;
#3996=LINE ( 'NONE', #2504, #3558 ) ;
#3998=CARTESIAN_POINT ( 'NONE',  ( 0.000000000000000000, -9.999999999999998224, 5.750000000000000000 ) ) ;
#4012=EDGE_CURVE ( 'NONE', #2074, #7471, #6987, .T. ) ;
#4017=ORIENTED_EDGE ( 'NONE', *, *, #4628, .F. ) ;
#4018=CARTESIAN_POINT ( 'NONE',  ( 5.114683531250000748, -29.35937500034139802, 0.000000000000000000 ) ) ;
#4020=DIRECTION ( 'NONE',  ( 0.000000000000000000, 1.000000000000000000, 0.000000000000000000 ) ) ;
#4021=CARTESIAN_POINT ( 'NONE',  ( -2.557341765624999042, -27.08854166700806232, -4.429445870380400052 ) ) ;
#4025=CARTESIAN_POINT ( 'NONE',  ( 2.557341765625000818, -27.06770833367473017, -4.429445870380400052 ) ) ;
#4026=CARTESIAN_POINT ( 'NONE',  ( 0.000000000000000000, 0.000000000000000000, 0.000000000000000000 ) ) ;
#4027=EDGE_CURVE ( 'NONE', #5643, #8929, #8512, .T. ) ;
#4028=CARTESIAN_POINT ( 'NONE',  ( 2.557341765624996821, -29.46354166700806232, 4.429445870380401828 ) ) ;
#4031=FACE_OUTER_BOUND ( 'NONE', #6432, .T. ) ;
#4040=CARTESIAN_POINT ( 'NONE',  ( 2.625000000000000444, -28.48958333401612819, -4.546633369868303021 ) ) ;
#4042=ORIENTED_EDGE ( 'NONE', *, *, #3134, .F. ) ;
#4045=CARTESIAN_POINT ( 'NONE',  ( 6.972266317189433020E-16, -29.43750000000000000, -5.250000000000000000 ) ) ;
#4053=CARTESIAN_POINT ( 'NONE',  ( 0.000000000000000000, -30.00000000000000000, 5.250000000000000000 ) ) ;
#4057=CARTESIAN_POINT ( 'NONE',  ( -1.406733260263385521, -27.10491455036742536, 5.250000000000006217 ) ) ;
#4058=CARTESIAN_POINT ( 'NONE',  ( 5.182341765625000818, -26.96093750017070079, 0.000000000000000000 ) ) ;
#4063=CARTESIAN_POINT ( 'NONE',  ( -2.557341765625002594, -28.19270833367473017, 4.429445870380399164 ) ) ;
#4066=CARTESIAN_POINT ( 'NONE',  ( -5.114683531249999859, -28.06770833367473017, -2.952963913586935440 ) ) ;
#4068=ADVANCED_FACE ( 'NONE', ( #5018 ), #7314, .T. ) ;
#4069=CARTESIAN_POINT ( 'NONE',  ( 1.185285273922203525E-14, -28.96875000068279959, -5.249999999999999112 ) ) ;
#4070=CARTESIAN_POINT ( 'NONE',  ( 2.300847884672513123E-14, -28.43750000000000000, -5.250000000000000000 ) ) ;
#4071=CARTESIAN_POINT ( 'NONE',  ( -5.114683531250000748, -29.02604166700806587, 2.952963913586931888 ) ) ;
#4072=ADVANCED_FACE ( 'NONE', ( #2906 ), #8567, .T. ) ;
#4077=DIRECTION ( 'NONE',  ( 0.000000000000000000, 0.000000000000000000, 1.000000000000000000 ) ) ;
#4081=ORIENTED_EDGE ( 'NONE', *, *, #1054, .T. ) ;
#4082=EDGE_CURVE ( 'NONE', #8842, #3705, #5116, .T. ) ;
#4084=CARTESIAN_POINT ( 'NONE',  ( 5.250000000000000000, -28.28125000068279604, 0.000000000000000000 ) ) ;
#4090=FACE_OUTER_BOUND ( 'NONE', #3004, .T. ) ;
#4091=PLANE ( 'NONE',  #4935 ) ;
#4094=CARTESIAN_POINT ( 'NONE',  ( 2.033577675846918216E-14, -27.59375000068279959, 5.250000000000000888 ) ) ;
#4097=EDGE_CURVE ( 'NONE', #7275, #3705, #3033, .T. ) ;
#4103=CARTESIAN_POINT ( 'NONE',  ( 0.000000000000000000, -9.999999999999998224, 0.000000000000000000 ) ) ;
#4104=CARTESIAN_POINT ( 'NONE',  ( 0.000000000000000000, -30.00000000000000000, 0.000000000000000000 ) ) ;
#4107=CARTESIAN_POINT ( 'NONE',  ( -5.114683531250000748, -27.25520833367473017, -2.952963913586935440 ) ) ;
#4110=CARTESIAN_POINT ( 'NONE',  ( -2.624999999999998668, -29.91666666666666430, -4.546633369868303021 ) ) ;
#4112=CARTESIAN_POINT ( 'NONE',  ( -2.557341765624999042, -29.58854166700806232, -4.429445870380400052 ) ) ;
#4113=CARTESIAN_POINT ( 'NONE',  ( 5.114683531249998971, -28.94270833367473017, 2.952963913586936329 ) ) ;
#4117=CARTESIAN_POINT ( 'NONE',  ( -1.975475456537005874E-15, -28.84375000068279959, 5.250000000000000000 ) ) ;
#4123=CARTESIAN_POINT ( 'NONE',  ( -5.114683531250000748, -29.48437500034139802, -6.263680815196995234E-16 ) ) ;
#4126=ORIENTED_EDGE ( 'NONE', *, *, #905, .T. ) ;
#4129=CARTESIAN_POINT ( 'NONE',  ( 0.000000000000000000, -30.00000000000000000, 0.000000000000000000 ) ) ;
#4132=CARTESIAN_POINT ( 'NONE',  ( 5.182341765625000818, -26.96093750017070079, 0.000000000000000000 ) ) ;
#4135=CARTESIAN_POINT ( 'NONE',  ( -2.557341765625002594, -28.44270833367473017, 4.429445870380399164 ) ) ;
#4138=EDGE_CURVE ( 'NONE', #8220, #2054, #8303, .T. ) ;
#4145=CARTESIAN_POINT ( 'NONE',  ( 0.000000000000000000, -30.00000000000000000, 5.250000000000000000 ) ) ;
#4147=VERTEX_POINT ( 'NONE', #789 ) ;
#4149=VECTOR ( 'NONE', #4904, 1000.000000000000000 ) ;
#4150=CARTESIAN_POINT ( 'NONE',  ( -5.114683531250001636, -27.71354166700806587, 2.952963913586931444 ) ) ;
#4152=CARTESIAN_POINT ( 'NONE',  ( 3.616337804771879580E-16, -27.35937500034140157, -5.905927827173866440 ) ) ;
#4153=CYLINDRICAL_SURFACE ( 'NONE', #3190, 4.250000000000000000 ) ;
#4154=CARTESIAN_POINT ( 'NONE',  ( -2.557341765625002594, -28.75520833367473017, 4.429445870380399164 ) ) ;
#4158=CARTESIAN_POINT ( 'NONE',  ( -2.557341765625002594, -28.75520833367473017, 4.429445870380399164 ) ) ;
#4161=ADVANCED_FACE ( 'NONE', ( #8698 ), #881, .T. ) ;
#4163=LINE ( 'NONE', #100, #8380 ) ;
#4170=CARTESIAN_POINT ( 'NONE',  ( -2.557341765624999042, -29.27604166700806232, -4.429445870380400052 ) ) ;
#4172=ORIENTED_EDGE ( 'NONE', *, *, #5831, .F. ) ;
#4177=CARTESIAN_POINT ( 'NONE',  ( -1.406733260263382856, -27.67633545031536713, -5.250000000000006217 ) ) ;
#4181=CARTESIAN_POINT ( 'NONE',  ( 5.114683531249998971, -28.63020833367472662, 2.952963913586936329 ) ) ;
#4188=CARTESIAN_POINT ( 'NONE',  ( 5.249999999999999112, -28.97916666666666430, -3.031088913245534755 ) ) ;
#4189=( NAMED_UNIT ( * ) SI_UNIT ( $, .STERADIAN. ) SOLID_ANGLE_UNIT ( ) );
#4195=CARTESIAN_POINT ( 'NONE',  ( -5.114683531250000748, -27.00520833367473017, -2.952963913586935440 ) ) ;
#4197=CARTESIAN_POINT ( 'NONE',  ( -5.114683531250000748, -28.04687500034139802, -6.263680815196995234E-16 ) ) ;
#4200=CARTESIAN_POINT ( 'NONE',  ( 3.616337804771879580E-16, -28.85937500034139802, -5.905927827173866440 ) ) ;
#4202=CARTESIAN_POINT ( 'NONE',  ( 2.557341765624996821, -28.21354166700806587, 4.429445870380401828 ) ) ;
#4203=CARTESIAN_POINT ( 'NONE',  ( -2.324088772396477476E-15, -29.68750000000000000, -5.250000000000000000 ) ) ;
#4205=CARTESIAN_POINT ( 'NONE',  ( 5.204748896376250699E-16, -9.999999999999998224, -4.250000000000000000 ) ) ;
#4206=CARTESIAN_POINT ( 'NONE',  ( 0.000000000000000000, -9.000000000000000000, 5.750000000000000000 ) ) ;
#4207=AXIS2_PLACEMENT_3D ( 'NONE', #5946, #8786, #2416 ) ;
#4215=CARTESIAN_POINT ( 'NONE',  ( -5.250000000000000888, -27.13541666734946389, 3.031088913245532979 ) ) ;
#4216=VECTOR ( 'NONE', #5336, 1000.000000000000000 ) ;
#4226=CARTESIAN_POINT ( 'NONE',  ( -5.114683531250000748, -29.23437500034139802, -6.263680815196995234E-16 ) ) ;
#4231=CARTESIAN_POINT ( 'NONE',  ( 0.000000000000000000, -30.00000000000000000, 0.000000000000000000 ) ) ;
#4235=PLANE ( 'NONE',  #7884 ) ;
#4236=CARTESIAN_POINT ( 'NONE',  ( -5.249999999999999112, -26.92708333401612819, -3.031088913245536975 ) ) ;
#4237=ADVANCED_FACE ( 'NONE', ( #1450 ), #4251, .F. ) ;
#4240=CARTESIAN_POINT ( 'NONE',  ( -2.557341765625002594, -27.19270833367473017, 4.429445870380399164 ) ) ;
#4242=CARTESIAN_POINT ( 'NONE',  ( 3.712013335537174572E-16, -29.68750000000000000, -6.062177826491070398 ) ) ;
#4244=CARTESIAN_POINT ( 'NONE',  ( -5.114683531250001636, -29.02604166700806587, 2.952963913586931444 ) ) ;
#4245=CARTESIAN_POINT ( 'NONE',  ( 5.114683531249998971, -27.19270833367473017, 2.952963913586936329 ) ) ;
#4246=CARTESIAN_POINT ( 'NONE',  ( -5.250000000000000000, -28.40625000068279604, -6.429395695523604153E-16 ) ) ;
#4249=DIRECTION ( 'NONE',  ( 0.000000000000000000, 0.000000000000000000, 1.000000000000000000 ) ) ;
#4251=PLANE ( 'NONE',  #4502 ) ;
#4252=CARTESIAN_POINT ( 'NONE',  ( -1.975475456537005874E-15, -29.59375000068279249, 5.250000000000000000 ) ) ;
#4254=ORIENTED_EDGE ( 'NONE', *, *, #5831, .T. ) ;
#4255=CARTESIAN_POINT ( 'NONE',  ( 5.249999999999999112, -27.30208333401612819, 3.031088913245538308 ) ) ;
#4261=VERTEX_POINT ( 'NONE', #3511 ) ;
#4266=CARTESIAN_POINT ( 'NONE',  ( -5.114683531250000748, -28.46354166700806587, 2.952963913586931888 ) ) ;
#4268=CARTESIAN_POINT ( 'NONE',  ( 5.250000000000000000, -29.03125000068279604, 0.000000000000000000 ) ) ;
#4271=( BOUNDED_CURVE ( )  B_SPLINE_CURVE ( 2, ( #2157, #7832, #2111, #4893, #5555, #6295, #6423, #7131, #753 ),
 .UNSPECIFIED., .F., .T. ) 
 B_SPLINE_CURVE_WITH_KNOTS ( ( 3, 2, 2, 2, 3 ),
 ( 0.4791666666666666852, 0.4861111111111111049, 0.5000000000000000000, 0.5138888888888888395, 0.5208333333333332593 ),
 .UNSPECIFIED. ) 
 CURVE ( )  GEOMETRIC_REPRESENTATION_ITEM ( )  RATIONAL_B_SPLINE_CURVE ( ( 0.9330127018922194093, 0.9330127018922196314, 1.000000000000000000, 0.8660254037844387076, 1.000000000000000000, 0.8660254037844387076, 1.000000000000000000, 0.9330127018922198534, 0.9330127018922192983 ) ) 
 REPRESENTATION_ITEM ( '' )  );
#4280=ORIENTED_EDGE ( 'NONE', *, *, #5363, .F. ) ;
#4286=CARTESIAN_POINT ( 'NONE',  ( -5.250000000000000000, -29.62500000000000000, -6.429395695523604153E-16 ) ) ;
#4288=CARTESIAN_POINT ( 'NONE',  ( 2.557341765625000818, -29.13020833367473017, -4.429445870380400052 ) ) ;
#4290=CARTESIAN_POINT ( 'NONE',  ( -5.114683531249999859, -27.56770833367473017, -2.952963913586935440 ) ) ;
#4295=CARTESIAN_POINT ( 'NONE',  ( 5.114683531250000748, -29.92187500034139802, 0.000000000000000000 ) ) ;
#4301=CARTESIAN_POINT ( 'NONE',  ( 5.250000000000000000, -27.01041666734946389, -3.031088913245534755 ) ) ;
#4304=ORIENTED_EDGE ( 'NONE', *, *, #4479, .T. ) ;
#4308=FACE_BOUND ( 'NONE', #4309, .T. ) ;
#4309=EDGE_LOOP ( 'NONE', ( #2941, #2473 ) ) ;
#4314=CARTESIAN_POINT ( 'NONE',  ( -5.114683531250000748, -28.98437500034139802, -6.263680815196995234E-16 ) ) ;
#4315=CARTESIAN_POINT ( 'NONE',  ( 5.249999999999999112, -27.51041666734946389, -3.031088913245534755 ) ) ;
#4322=CARTESIAN_POINT ( 'NONE',  ( 2.033577675846918216E-14, -27.31250000000000000, 5.250000000000000888 ) ) ;
#4324=CARTESIAN_POINT ( 'NONE',  ( -1.406733260263385521, -27.60491455036742181, 5.250000000000006217 ) ) ;
#4326=( BOUNDED_CURVE ( )  B_SPLINE_CURVE ( 2, ( #6482, #8632, #8816, #4402, #5231, #8076, #7232, #1753, #1605 ),
 .UNSPECIFIED., .F., .T. ) 
 B_SPLINE_CURVE_WITH_KNOTS ( ( 3, 2, 2, 2, 3 ),
 ( 0.02083333333333333218, 0.02777777777777777624, 0.04166666666666666435, 0.05555555555555555247, 0.06250000000000000000 ),
 .UNSPECIFIED. ) 
 CURVE ( )  GEOMETRIC_REPRESENTATION_ITEM ( )  RATIONAL_B_SPLINE_CURVE ( ( 0.9330127018922194093, 0.9330127018922194093, 1.000000000000000000, 0.8660254037844387076, 1.000000000000000000, 0.8660254037844387076, 1.000000000000000000, 0.9330127018922194093, 0.9330127018922194093 ) ) 
 REPRESENTATION_ITEM ( '' )  );
#4329=CARTESIAN_POINT ( 'NONE',  ( -2.557341765625002594, -26.94270833367473017, 4.429445870380399164 ) ) ;
#4333=CARTESIAN_POINT ( 'NONE',  ( -2.624999999999998668, -28.66666666666666785, -4.546633369868303021 ) ) ;
#4335=CARTESIAN_POINT ( 'NONE',  ( -1.084901341431563726E-15, -28.23437500034139447, 5.905927827173866440 ) ) ;
#4336=CARTESIAN_POINT ( 'NONE',  ( 5.114683531249999859, -28.15104166700806587, -2.952963913586932776 ) ) ;
#4338=DIRECTION ( 'NONE',  ( 0.000000000000000000, 1.000000000000000000, 0.000000000000000000 ) ) ;
#4339=CYLINDRICAL_SURFACE ( 'NONE', #1628, 5.250000000000000000 ) ;
#4341=CARTESIAN_POINT ( 'NONE',  ( 2.557341765624996821, -29.71354166700806232, 4.429445870380401828 ) ) ;
#4345=CARTESIAN_POINT ( 'NONE',  ( -5.250000000000000000, -28.65625000068279604, -6.429395695523604153E-16 ) ) ;
#4347=CARTESIAN_POINT ( 'NONE',  ( 5.114683531249998971, -27.88020833367473017, 2.952963913586936329 ) ) ;
#4348=EDGE_CURVE ( 'NONE', #8645, #8220, #4271, .T. ) ;
#4350=VERTEX_POINT ( 'NONE', #3598 ) ;
#4357=ORIENTED_EDGE ( 'NONE', *, *, #1575, .T. ) ;
#4358=LINE ( 'NONE', #6349, #467 ) ;
#4359=CARTESIAN_POINT ( 'NONE',  ( 5.249999999999999112, -29.30208333401613174, 3.031088913245538308 ) ) ;
#4362=CARTESIAN_POINT ( 'NONE',  ( -1.084901341431563923E-15, -27.42187500034139802, 5.905927827173866440 ) ) ;
#4363=DIRECTION ( 'NONE',  ( 0.000000000000000000, 1.000000000000000000, 0.000000000000000000 ) ) ;
#4378=VERTEX_POINT ( 'NONE', #8489 ) ;
#4379=CARTESIAN_POINT ( 'NONE',  ( 2.624999999999996891, -29.29166666666666785, 4.546633369868304797 ) ) ;
#4381=CARTESIAN_POINT ( 'NONE',  ( 5.114683531250000748, -28.40104166700806587, -2.952963913586932776 ) ) ;
#4383=CARTESIAN_POINT ( 'NONE',  ( 5.114683531249998971, -27.94270833367473017, 2.952963913586936329 ) ) ;
#4388=CARTESIAN_POINT ( 'NONE',  ( -2.625000000000002220, -27.36458333401612819, 4.546633369868302132 ) ) ;
#4389=FACE_OUTER_BOUND ( 'NONE', #3284, .T. ) ;
#4394=CARTESIAN_POINT ( 'NONE',  ( 2.557341765624996821, -28.90104166700806587, 4.429445870380401828 ) ) ;
#4397=DIRECTION ( 'NONE',  ( 0.000000000000000000, 1.000000000000000000, 0.000000000000000000 ) ) ;
#4399=CARTESIAN_POINT ( 'NONE',  ( 2.624999999999996891, -27.54166666666666430, 4.546633369868304797 ) ) ;
#4402=CARTESIAN_POINT ( 'NONE',  ( -5.249999999999999112, -29.89583333333333215, -3.031088913245536975 ) ) ;
#4403=CARTESIAN_POINT ( 'NONE',  ( 5.250000000000000000, -29.26041666734946389, -3.031088913245534755 ) ) ;
#4406=CARTESIAN_POINT ( 'NONE',  ( 2.557341765624996821, -27.40104166700806587, 4.429445870380401828 ) ) ;
#4407=CARTESIAN_POINT ( 'NONE',  ( 0.000000000000000000, -30.00000000000000000, 5.250000000000000000 ) ) ;
#4408=CARTESIAN_POINT ( 'NONE',  ( 0.000000000000000000, -9.999999999999998224, 0.000000000000000000 ) ) ;
#4415=CARTESIAN_POINT ( 'NONE',  ( -2.625000000000002220, -27.83333333333333215, 4.546633369868302132 ) ) ;
#4425=CARTESIAN_POINT ( 'NONE',  ( 3.712013335537174572E-16, -29.43750000000000000, -6.062177826491070398 ) ) ;
#4426=CARTESIAN_POINT ( 'NONE',  ( 2.557341765624996821, -27.71354166700806587, 4.429445870380401828 ) ) ;
#4431=CARTESIAN_POINT ( 'NONE',  ( -5.249999999999999112, -27.42708333401612819, -3.031088913245536975 ) ) ;
#4432=CARTESIAN_POINT ( 'NONE',  ( 5.114683531249998971, -29.69270833367473017, 2.952963913586936329 ) ) ;
#4436=CARTESIAN_POINT ( 'NONE',  ( -1.975475456537005874E-15, -28.84375000068279959, 5.249999999999999112 ) ) ;
#4437=CARTESIAN_POINT ( 'NONE',  ( 5.114683531250000748, -28.35937500034139447, 0.000000000000000000 ) ) ;
#4439=ORIENTED_EDGE ( 'NONE', *, *, #3553, .T. ) ;
#4440=DIRECTION ( 'NONE',  ( 0.000000000000000000, 1.000000000000000000, 0.000000000000000000 ) ) ;
#4446=CARTESIAN_POINT ( 'NONE',  ( 2.625000000000000444, -29.48958333401613174, -4.546633369868303021 ) ) ;
#4448=CARTESIAN_POINT ( 'NONE',  ( 3.616337804771879580E-16, -27.54687500034140157, -5.905927827173866440 ) ) ;
#4449=CARTESIAN_POINT ( 'NONE',  ( 2.300847884672513123E-14, -27.46875000068279604, -5.250000000000000000 ) ) ;
#4452=( GEOMETRIC_REPRESENTATION_CONTEXT ( 3 ) GLOBAL_UNCERTAINTY_ASSIGNED_CONTEXT ( ( #345 ) ) GLOBAL_UNIT_ASSIGNED_CONTEXT ( ( #5708, #8552, #4189 ) ) REPRESENTATION_CONTEXT ( 'NONE', 'WORKASPACE' ) );
#4460=EDGE_CURVE ( 'NONE', #3057, #6454, #3544, .T. ) ;
#4462=ORIENTED_EDGE ( 'NONE', *, *, #1859, .F. ) ;
#4470=CARTESIAN_POINT ( 'NONE',  ( -1.113604000661152470E-15, -27.31250000000000000, 6.062177826491070398 ) ) ;
#4472=CARTESIAN_POINT ( 'NONE',  ( 5.114683531250000748, -27.65104166700806587, -2.952963913586932776 ) ) ;
#4473=AXIS2_PLACEMENT_3D ( 'NONE', #5332, #1907, #3395 ) ;
#4476=DIRECTION ( 'NONE',  ( 0.000000000000000000, 0.000000000000000000, 1.000000000000000000 ) ) ;
#4478=EDGE_CURVE ( 'NONE', #7180, #4261, #5218, .T. ) ;
#4479=EDGE_CURVE ( 'NONE', #3341, #5696, #2005, .T. ) ;
#4481=CARTESIAN_POINT ( 'NONE',  ( 5.249999999999999112, -28.72916666666666785, -3.031088913245534755 ) ) ;
#4482=CARTESIAN_POINT ( 'NONE',  ( 5.114683531249999859, -29.40104166700806232, -2.952963913586932776 ) ) ;
#4487=CARTESIAN_POINT ( 'NONE',  ( 6.972266317189433020E-16, -27.93749999999999289, -5.250000000000000000 ) ) ;
#4488=CARTESIAN_POINT ( 'NONE',  ( -2.557341765624999042, -28.52604166700806587, -4.429445870380400052 ) ) ;
#4490=ORIENTED_EDGE ( 'NONE', *, *, #672, .T. ) ;
#4495=CARTESIAN_POINT ( 'NONE',  ( -2.625000000000002220, -29.08333333333333215, 4.546633369868302132 ) ) ;
#4497=( BOUNDED_CURVE ( )  B_SPLINE_CURVE ( 2, ( #8628, #1655, #4399, #3062, #1602, #5882, #907, #3754, #6580 ),
 .UNSPECIFIED., .F., .F. ) 
 B_SPLINE_CURVE_WITH_KNOTS ( ( 3, 2, 2, 2, 3 ),
 ( 0.8125000000000000000, 0.8194444444444444198, 0.8333333333333333703, 0.8472222222222222099, 0.8541666666666666297 ),
 .UNSPECIFIED. ) 
 CURVE ( )  GEOMETRIC_REPRESENTATION_ITEM ( )  RATIONAL_B_SPLINE_CURVE ( ( 0.9330127018922194093, 0.9330127018922194093, 1.000000000000000000, 0.8660254037844387076, 1.000000000000000000, 0.8660254037844387076, 1.000000000000000000, 0.9330127018922198534, 0.9330127018922192983 ) ) 
 REPRESENTATION_ITEM ( '' )  );
#4499=CARTESIAN_POINT ( 'NONE',  ( 2.624999999999996891, -29.07291666734946389, 4.546633369868304797 ) ) ;
#4501=CARTESIAN_POINT ( 'NONE',  ( 5.114683531250000748, -27.85937500034139802, 0.000000000000000000 ) ) ;
#4502=AXIS2_PLACEMENT_3D ( 'NONE', #4977, #7084, #16 ) ;
#4506=CARTESIAN_POINT ( 'NONE',  ( 0.000000000000000000, -9.999999999999998224, 0.000000000000000000 ) ) ;
#4518=DIRECTION ( 'NONE',  ( 0.000000000000000000, 0.000000000000000000, 1.000000000000000000 ) ) ;
#4519=ORIENTED_EDGE ( 'NONE', *, *, #4478, .F. ) ;
#4523=CARTESIAN_POINT ( 'NONE',  ( 5.250000000000000000, -28.24999999999999645, 0.000000000000000000 ) ) ;
#4529=CARTESIAN_POINT ( 'NONE',  ( 2.624999999999996891, -28.82291666734946389, 4.546633369868304797 ) ) ;
#4531=CARTESIAN_POINT ( 'NONE',  ( -5.114683531249999859, -28.56770833367473017, -2.952963913586935440 ) ) ;
#4532=CARTESIAN_POINT ( 'NONE',  ( 2.625000000000000444, -28.23958333401612819, -4.546633369868303021 ) ) ;
#4535=CARTESIAN_POINT ( 'NONE',  ( 2.557341765625000818, -28.56770833367473017, -4.429445870380400052 ) ) ;
#4536=ORIENTED_EDGE ( 'NONE', *, *, #3417, .T. ) ;
#4544=CARTESIAN_POINT ( 'NONE',  ( -2.624999999999998668, -28.69791666734946389, -4.546633369868303021 ) ) ;
#4546=CARTESIAN_POINT ( 'NONE',  ( 5.114683531249998971, -27.13020833367473372, 2.952963913586936329 ) ) ;
#4551=SHAPE_REPRESENTATION ( 'outer body', ( #888 ), #6342 ) ;
#4558=EDGE_CURVE ( 'NONE', #3585, #7800, #8296, .T. ) ;
#4560=CARTESIAN_POINT ( 'NONE',  ( -5.250000000000000888, -29.60416666666666430, 3.031088913245533423 ) ) ;
#4564=ORIENTED_EDGE ( 'NONE', *, *, #5081, .F. ) ;
#4565=CARTESIAN_POINT ( 'NONE',  ( 2.624999999999996891, -28.29166666666666785, 4.546633369868304797 ) ) ;
#4569=CARTESIAN_POINT ( 'NONE',  ( -5.250000000000000000, -29.40625000068279604, -6.429395695523604153E-16 ) ) ;
#4571=CARTESIAN_POINT ( 'NONE',  ( -2.557341765624999042, -29.52604166700806232, -4.429445870380400052 ) ) ;
#4574=CARTESIAN_POINT ( 'NONE',  ( -5.250000000000000000, -28.12499999999999645, -6.429395695523604153E-16 ) ) ;
#4575=CARTESIAN_POINT ( 'NONE',  ( -2.557341765625002594, -29.00520833367473017, 4.429445870380399164 ) ) ;
#4578=ORIENTED_EDGE ( 'NONE', *, *, #8719, .F. ) ;
#4579=CARTESIAN_POINT ( 'NONE',  ( -5.250000000000000888, -27.88541666734946389, 3.031088913245533423 ) ) ;
#4580=CARTESIAN_POINT ( 'NONE',  ( -2.557341765625002594, -27.19270833367473017, 4.429445870380399164 ) ) ;
#4582=CARTESIAN_POINT ( 'NONE',  ( 2.300847884672513123E-14, -27.43750000000000355, -5.250000000000000000 ) ) ;
#4588=ADVANCED_FACE ( 'NONE', ( #478 ), #3324, .T. ) ;
#4590=CARTESIAN_POINT ( 'NONE',  ( -5.250000000000000000, -27.67708333401612464, -3.031088913245536531 ) ) ;
#4597=PRODUCT ( 'outer body', 'outer body', '', ( #3400 ) ) ;
#4601=CARTESIAN_POINT ( 'NONE',  ( 2.625000000000000444, -29.70833333333333215, -4.546633369868303021 ) ) ;
#4606=DIRECTION ( 'NONE',  ( 0.000000000000000000, 0.000000000000000000, 1.000000000000000000 ) ) ;
#4612=CARTESIAN_POINT ( 'NONE',  ( -2.624999999999998668, -27.91666666666666430, -4.546633369868303021 ) ) ;
#4614=VERTEX_POINT ( 'NONE', #1033 ) ;
#4615=CARTESIAN_POINT ( 'NONE',  ( 5.114683531250000748, -26.92187500034139802, 0.000000000000000000 ) ) ;
#4616=AXIS2_PLACEMENT_3D ( 'NONE', #1525, #733, #7065 ) ;
#4618=CARTESIAN_POINT ( 'NONE',  ( -5.114683531250001636, -28.96354166700807298, 2.952963913586931444 ) ) ;
#4622=CARTESIAN_POINT ( 'NONE',  ( -2.557341765624999042, -28.08854166700806587, -4.429445870380400052 ) ) ;
#4624=CARTESIAN_POINT ( 'NONE',  ( -5.114683531249999859, -27.50520833367472662, -2.952963913586935440 ) ) ;
#4625=ORIENTED_EDGE ( 'NONE', *, *, #7129, .T. ) ;
#4628=EDGE_CURVE ( 'NONE', #849, #4614, #2632, .T. ) ;
#4630=CARTESIAN_POINT ( 'NONE',  ( -1.975475456537005874E-15, -29.09375000068278894, 5.250000000000000000 ) ) ;
#4635=CARTESIAN_POINT ( 'NONE',  ( 3.712013335537174572E-16, -27.46875000068279959, -6.062177826491070398 ) ) ;
#4637=ADVANCED_FACE ( 'NONE', ( #4667 ), #4757, .T. ) ;
#4641=ADVANCED_BREP_SHAPE_REPRESENTATION ( '', ( #2131, #888 ), #6342 ) ;
#4645=VECTOR ( 'NONE', #239, 1000.000000000000000 ) ;
#4646=CARTESIAN_POINT ( 'NONE',  ( 5.114683531249999859, -29.58854166700806232, -2.952963913586932776 ) ) ;
#4647=CARTESIAN_POINT ( 'NONE',  ( 5.249999999999997335, -27.77083333333333215, 3.031088913245538308 ) ) ;
#4654=CARTESIAN_POINT ( 'NONE',  ( 5.249999999999999112, -27.77083333333333215, 3.031088913245538308 ) ) ;
#4655=DIRECTION ( 'NONE',  ( 0.000000000000000000, 1.000000000000000000, 0.000000000000000000 ) ) ;
#4656=CARTESIAN_POINT ( 'NONE',  ( 5.114683531250000748, -27.15104166700806587, -2.952963913586932776 ) ) ;
#4664=CARTESIAN_POINT ( 'NONE',  ( -2.557341765624999042, -29.02604166700806587, -4.429445870380400052 ) ) ;
#4667=FACE_OUTER_BOUND ( 'NONE', #7053, .T. ) ;
#4668=CARTESIAN_POINT ( 'NONE',  ( 5.114683531250000748, -28.42187500034139802, 0.000000000000000000 ) ) ;
#4671=CARTESIAN_POINT ( 'NONE',  ( 2.557341765624996821, -26.90104166700806232, 4.429445870380401828 ) ) ;
#4676=CARTESIAN_POINT ( 'NONE',  ( -2.625000000000002220, -28.58333333333333215, 4.546633369868302132 ) ) ;
#4680=VERTEX_POINT ( 'NONE', #7459 ) ;
#4682=CARTESIAN_POINT ( 'NONE',  ( 2.625000000000000444, -27.98958333401612819, -4.546633369868303021 ) ) ;
#4688=ADVANCED_FACE ( 'NONE', ( #3187 ), #7506, .T. ) ;
#4689=CARTESIAN_POINT ( 'NONE',  ( 5.250000000000000000, -28.24999999999999645, 0.000000000000000000 ) ) ;
#4692=DIRECTION ( 'NONE',  ( 0.000000000000000000, 1.000000000000000000, 0.000000000000000000 ) ) ;
#4701=CARTESIAN_POINT ( 'NONE',  ( 2.624999999999996891, -29.04166666666666785, 4.546633369868304797 ) ) ;
#4709=CARTESIAN_POINT ( 'NONE',  ( -2.557341765625002594, -28.69270833367473017, 4.429445870380399164 ) ) ;
#4712=CARTESIAN_POINT ( 'NONE',  ( 5.114683531249998971, -27.69270833367472662, 2.952963913586936329 ) ) ;
#4713=CYLINDRICAL_SURFACE ( 'NONE', #9112, 5.250000000000000000 ) ;
#4715=CARTESIAN_POINT ( 'NONE',  ( 5.114683531250000748, -27.10937500034139802, 0.000000000000000000 ) ) ;
#4716=CARTESIAN_POINT ( 'NONE',  ( -5.114683531250000748, -29.04687500034139802, -6.263680815196995234E-16 ) ) ;
#4718=DIRECTION ( 'NONE',  ( 0.000000000000000000, 0.000000000000000000, 1.000000000000000000 ) ) ;
#4720=CARTESIAN_POINT ( 'NONE',  ( -5.249999999999999112, -29.17708333401613174, -3.031088913245536975 ) ) ;
#4721=LINE ( 'NONE', #7562, #732 ) ;
#4724=ORIENTED_EDGE ( 'NONE', *, *, #5158, .F. ) ;
#4725=DIRECTION ( 'NONE',  ( 0.000000000000000000, 0.000000000000000000, 1.000000000000000000 ) ) ;
#4726=CARTESIAN_POINT ( 'NONE',  ( -5.250000000000000888, -27.38541666734946389, 3.031088913245532979 ) ) ;
#4729=ORIENTED_EDGE ( 'NONE', *, *, #362, .F. ) ;
#4736=CARTESIAN_POINT ( 'NONE',  ( -2.557341765624999042, -29.77604166700806232, -4.429445870380400052 ) ) ;
#4737=ORIENTED_EDGE ( 'NONE', *, *, #191, .T. ) ;
#4745=CARTESIAN_POINT ( 'NONE',  ( -1.406733260263382856, -27.20758545099817027, -5.250000000000006217 ) ) ;
#4748=EDGE_CURVE ( 'NONE', #7800, #1439, #5077, .T. ) ;
#4755=CARTESIAN_POINT ( 'NONE',  ( -1.084901341431563726E-15, -29.17187500034139802, 5.905927827173866440 ) ) ;
#4757=CYLINDRICAL_SURFACE ( 'NONE', #930, 5.250000000000000000 ) ;
#4758=CARTESIAN_POINT ( 'NONE',  ( 5.114683531249998971, -27.94270833367473017, 2.952963913586936329 ) ) ;
#4760=CARTESIAN_POINT ( 'NONE',  ( -5.114683531250000748, -27.48437500034139802, -6.263680815196995234E-16 ) ) ;
#4763=CARTESIAN_POINT ( 'NONE',  ( -2.557341765624999042, -28.83854166700806587, -4.429445870380400052 ) ) ;
#4767=CARTESIAN_POINT ( 'NONE',  ( 6.972266317189433020E-16, -29.93750000000000000, -5.250000000000000000 ) ) ;
#4771=ORIENTED_EDGE ( 'NONE', *, *, #3446, .T. ) ;
#4773=CARTESIAN_POINT ( 'NONE',  ( 5.249999999999999112, -27.80208333401612819, 3.031088913245538308 ) ) ;
#4777=ORIENTED_EDGE ( 'NONE', *, *, #756, .F. ) ;
#4781=CARTESIAN_POINT ( 'NONE',  ( 2.624999999999996891, -28.29166666666666785, 4.546633369868304797 ) ) ;
#4784=DIRECTION ( 'NONE',  ( 0.000000000000000000, 1.000000000000000000, 0.000000000000000000 ) ) ;
#4791=CARTESIAN_POINT ( 'NONE',  ( 2.033577675846918216E-14, -27.09375000068279604, 5.250000000000000888 ) ) ;
#4793=( BOUNDED_SURFACE ( )  B_SPLINE_SURFACE ( 1, 2, ( 
 ( #3954, #5478, #1814, #8277, #4736, #8829, #8325, #2509, #7626, #555, #407, #1767, #3398, #4646, #7440, #1064, #3909, #6731, #6834, #1114, #3212, #6031, #8869, #2564, #5383, #8234, #459, #6133, #6970, #8505, #4226, #2749, #9103, #3484, #4912, #4952, #5658, #2086, #6227, #598, #6310, #1471, #4314, #1294, #6352, #9187, #725, #7057, #5570, #639, #4826, #7760, #2883, #32, #5701, #681, #3528, #3443, #7149, #4181, #6269, #773, #7808, #5612, #2000, #8545, #6397, #4266, #4135, #2129, #2838, #1425, #1382, #7013, #7715, #7101, #9146, #3572, #5529, #2701, #2792, #8374, #2172, #4993, #7850, #8460, #9058, #7671, #8415, #2041, #4865, #1341, #6631, #6442, #2313, #3805, #4501, #5745, #861, #5935, #1708, #6588, #2217, #3068, #8587, #1661, #7286, #7982, #3110, #5794, #168, #4448, #8081, #216, #7943, #8681, #7194, #4362, #4406, #3018, #959, #1517, #8635, #7378, #3710, #2265, #5043, #7236, #3618, #259, #121, #4546, #8775, #7898, #2405, #5235, #76, #2926, #5093, #8030, #6486, #5887, #8726, #1564, #819 ),
 ( #6535, #3661, #5843, #2970, #5139, #1609, #912, #3759, #2358, #5188, #7333, #7691, #436, #6162, #5549, #3461, #485, #3851, #2061, #576, #1275, #6205, #4028, #9126, #8939, #3421, #1231, #8259, #2722, #2590, #3330, #1891, #6250, #8351, #6862, #8988, #7607, #9036, #9082, #8395, #2678, #1004, #4716, #4071, #5591, #8435, #5410, #4113, #6947, #4846, #1976, #2636, #4763, #7557, #5508, #6993, #4158, #619, #4806, #7650, #1183, #4888, #8302, #5457, #6810, #2020, #534, #6112, #6290, #1316, #2771, #1935, #3283, #6909, #3374, #56, #8525, #12, #5721, #4973, #6463, #7038, #4202, #2153, #662, #4336, #5017, #1542, #749, #3640, #2243, #2947, #7827, #6329, #3593, #4383, #1363, #6418, #7918, #8610, #3506, #1445, #838, #5819, #1493, #9165, #7171, #2814, #5768, #2195, #2905, #7214, #701, #4290, #8566, #2997, #796, #2860, #7873, #96, #5064, #3684, #6510, #146, #8658, #5678, #2289, #7740, #5634, #8484, #2106, #4245, #7125, #4931, #7787, #1406, #7079, #3549, #6370, #8153, #283, #3785, #192, #5911, #4615 ) ),
 .UNSPECIFIED., .F., .F., .F. ) 
 B_SPLINE_SURFACE_WITH_KNOTS ( ( 2, 2 ),
 ( 3, 2, 2, 2, 2, 2, 2, 2, 2, 2, 2, 2, 2, 2, 2, 2, 2, 2, 2, 2, 2, 2, 2, 2, 2, 2, 2, 2, 2, 2, 2, 2, 2, 2, 2, 2, 2, 2, 2, 2, 2, 2, 2, 2, 2, 2, 2, 2, 2, 2, 2, 2, 2, 2, 2, 2, 2, 2, 2, 2, 2, 2, 2, 2, 2, 2, 2, 2, 2, 2, 2, 2, 3 ),
 ( 0.000000000000000000, 1.000000000000000000 ),
 ( 0.000000000000000000, 0.01388888888888888812, 0.02777777777777777624, 0.04166666666666666435, 0.05555555555555555247, 0.06944444444444444753, 0.08333333333333332871, 0.09722222222222222376, 0.1111111111111111049, 0.1250000000000000000, 0.1388888888888888951, 0.1527777777777777901, 0.1666666666666666574, 0.1805555555555555525, 0.1944444444444444475, 0.2083333333333333426, 0.2222222222222222099, 0.2361111111111111049, 0.2500000000000000000, 0.2638888888888888951, 0.2777777777777777901, 0.2916666666666666852, 0.3055555555555555802, 0.3194444444444444198, 0.3333333333333333148, 0.3472222222222222099, 0.3611111111111111049, 0.3750000000000000000, 0.3888888888888888951, 0.4027777777777777901, 0.4166666666666666852, 0.4305555555555555802, 0.4444444444444444198, 0.4583333333333333148, 0.4722222222222222099, 0.4861111111111111049, 0.5000000000000000000, 0.5138888888888888395, 0.5277777777777777901, 0.5416666666666666297, 0.5555555555555555802, 0.5694444444444444198, 0.5833333333333333703, 0.5972222222222222099, 0.6111111111111111605, 0.6250000000000000000, 0.6388888888888888395, 0.6527777777777777901, 0.6666666666666666297, 0.6805555555555555802, 0.6944444444444444198, 0.7083333333333333703, 0.7222222222222222099, 0.7361111111111111605, 0.7500000000000000000, 0.7638888888888888395, 0.7777777777777777901, 0.7916666666666666297, 0.8055555555555555802, 0.8194444444444444198, 0.8333333333333333703, 0.8472222222222222099, 0.8611111111111111605, 0.8750000000000000000, 0.8888888888888888395, 0.9027777777777777901, 0.9166666666666666297, 0.9305555555555555802, 0.9444444444444444198, 0.9583333333333333703, 0.9722222222222222099, 0.9861111111111111605, 1.000000000000000000 ),
 .UNSPECIFIED. ) 
 GEOMETRIC_REPRESENTATION_ITEM ( )  RATIONAL_B_SPLINE_SURFACE ( (
 ( 1.000000000000000000, 0.8660254037844387076, 1.000000000000000000, 0.8660254037844387076, 1.000000000000000000, 0.8660254037844387076, 1.000000000000000000, 0.8660254037844387076, 1.000000000000000000, 0.8660254037844387076, 1.000000000000000000, 0.8660254037844387076, 1.000000000000000000, 0.8660254037844387076, 1.000000000000000000, 0.8660254037844387076, 1.000000000000000000, 0.8660254037844387076, 1.000000000000000000, 0.8660254037844387076, 1.000000000000000000, 0.8660254037844387076, 1.000000000000000000, 0.8660254037844387076, 1.000000000000000000, 0.8660254037844387076, 1.000000000000000000, 0.8660254037844387076, 1.000000000000000000, 0.8660254037844387076, 1.000000000000000000, 0.8660254037844387076, 1.000000000000000000, 0.8660254037844387076, 1.000000000000000000, 0.8660254037844387076, 1.000000000000000000, 0.8660254037844387076, 1.000000000000000000, 0.8660254037844387076, 1.000000000000000000, 0.8660254037844387076, 1.000000000000000000, 0.8660254037844387076, 1.000000000000000000, 0.8660254037844387076, 1.000000000000000000, 0.8660254037844387076, 1.000000000000000000, 0.8660254037844387076, 1.000000000000000000, 0.8660254037844387076, 1.000000000000000000, 0.8660254037844387076, 1.000000000000000000, 0.8660254037844387076, 1.000000000000000000, 0.8660254037844387076, 1.000000000000000000, 0.8660254037844387076, 1.000000000000000000, 0.8660254037844387076, 1.000000000000000000, 0.8660254037844387076, 1.000000000000000000, 0.8660254037844387076, 1.000000000000000000, 0.8660254037844387076, 1.000000000000000000, 0.8660254037844387076, 1.000000000000000000, 0.8660254037844387076, 1.000000000000000000, 0.8660254037844387076, 1.000000000000000000, 0.8660254037844387076, 1.000000000000000000, 0.8660254037844387076, 1.000000000000000000, 0.8660254037844387076, 1.000000000000000000, 0.8660254037844387076, 1.000000000000000000, 0.8660254037844387076, 1.000000000000000000, 0.8660254037844387076, 1.000000000000000000, 0.8660254037844387076, 1.000000000000000000, 0.8660254037844387076, 1.000000000000000000, 0.8660254037844387076, 1.000000000000000000, 0.8660254037844387076, 1.000000000000000000, 0.8660254037844387076, 1.000000000000000000, 0.8660254037844387076, 1.000000000000000000, 0.8660254037844387076, 1.000000000000000000, 0.8660254037844387076, 1.000000000000000000, 0.8660254037844387076, 1.000000000000000000, 0.8660254037844387076, 1.000000000000000000, 0.8660254037844387076, 1.000000000000000000, 0.8660254037844387076, 1.000000000000000000, 0.8660254037844387076, 1.000000000000000000, 0.8660254037844387076, 1.000000000000000000, 0.8660254037844387076, 1.000000000000000000, 0.8660254037844387076, 1.000000000000000000, 0.8660254037844387076, 1.000000000000000000, 0.8660254037844387076, 1.000000000000000000, 0.8660254037844387076, 1.000000000000000000, 0.8660254037844387076, 1.000000000000000000, 0.8660254037844387076, 1.000000000000000000, 0.8660254037844387076, 1.000000000000000000, 0.8660254037844387076, 1.000000000000000000, 0.8660254037844387076, 1.000000000000000000, 0.8660254037844387076, 1.000000000000000000, 0.8660254037844387076, 1.000000000000000000, 0.8660254037844387076, 1.000000000000000000, 0.8660254037844387076, 1.000000000000000000, 0.8660254037844387076, 1.000000000000000000),
 ( 1.000000000000000000, 0.8660254037844387076, 1.000000000000000000, 0.8660254037844387076, 1.000000000000000000, 0.8660254037844387076, 1.000000000000000000, 0.8660254037844387076, 1.000000000000000000, 0.8660254037844387076, 1.000000000000000000, 0.8660254037844387076, 1.000000000000000000, 0.8660254037844387076, 1.000000000000000000, 0.8660254037844387076, 1.000000000000000000, 0.8660254037844387076, 1.000000000000000000, 0.8660254037844387076, 1.000000000000000000, 0.8660254037844387076, 1.000000000000000000, 0.8660254037844387076, 1.000000000000000000, 0.8660254037844387076, 1.000000000000000000, 0.8660254037844387076, 1.000000000000000000, 0.8660254037844387076, 1.000000000000000000, 0.8660254037844387076, 1.000000000000000000, 0.8660254037844387076, 1.000000000000000000, 0.8660254037844387076, 1.000000000000000000, 0.8660254037844387076, 1.000000000000000000, 0.8660254037844387076, 1.000000000000000000, 0.8660254037844387076, 1.000000000000000000, 0.8660254037844387076, 1.000000000000000000, 0.8660254037844387076, 1.000000000000000000, 0.8660254037844387076, 1.000000000000000000, 0.8660254037844387076, 1.000000000000000000, 0.8660254037844387076, 1.000000000000000000, 0.8660254037844387076, 1.000000000000000000, 0.8660254037844387076, 1.000000000000000000, 0.8660254037844387076, 1.000000000000000000, 0.8660254037844387076, 1.000000000000000000, 0.8660254037844387076, 1.000000000000000000, 0.8660254037844387076, 1.000000000000000000, 0.8660254037844387076, 1.000000000000000000, 0.8660254037844387076, 1.000000000000000000, 0.8660254037844387076, 1.000000000000000000, 0.8660254037844387076, 1.000000000000000000, 0.8660254037844387076, 1.000000000000000000, 0.8660254037844387076, 1.000000000000000000, 0.8660254037844387076, 1.000000000000000000, 0.8660254037844387076, 1.000000000000000000, 0.8660254037844387076, 1.000000000000000000, 0.8660254037844387076, 1.000000000000000000, 0.8660254037844387076, 1.000000000000000000, 0.8660254037844387076, 1.000000000000000000, 0.8660254037844387076, 1.000000000000000000, 0.8660254037844387076, 1.000000000000000000, 0.8660254037844387076, 1.000000000000000000, 0.8660254037844387076, 1.000000000000000000, 0.8660254037844387076, 1.000000000000000000, 0.8660254037844387076, 1.000000000000000000, 0.8660254037844387076, 1.000000000000000000, 0.8660254037844387076, 1.000000000000000000, 0.8660254037844387076, 1.000000000000000000, 0.8660254037844387076, 1.000000000000000000, 0.8660254037844387076, 1.000000000000000000, 0.8660254037844387076, 1.000000000000000000, 0.8660254037844387076, 1.000000000000000000, 0.8660254037844387076, 1.000000000000000000, 0.8660254037844387076, 1.000000000000000000, 0.8660254037844387076, 1.000000000000000000, 0.8660254037844387076, 1.000000000000000000, 0.8660254037844387076, 1.000000000000000000, 0.8660254037844387076, 1.000000000000000000, 0.8660254037844387076, 1.000000000000000000, 0.8660254037844387076, 1.000000000000000000, 0.8660254037844387076, 1.000000000000000000, 0.8660254037844387076, 1.000000000000000000, 0.8660254037844387076, 1.000000000000000000, 0.8660254037844387076, 1.000000000000000000, 0.8660254037844387076, 1.000000000000000000, 0.8660254037844387076, 1.000000000000000000, 0.8660254037844387076, 1.000000000000000000) ) ) 
 REPRESENTATION_ITEM ( '' )  SURFACE ( )  );
#4798=CARTESIAN_POINT ( 'NONE',  ( -2.557341765625002594, -27.69270833367473017, 4.429445870380399164 ) ) ;
#4801=CARTESIAN_POINT ( 'NONE',  ( 2.625000000000000444, -29.95833333333333215, -4.546633369868303021 ) ) ;
#4804=CIRCLE ( 'NONE', #7632, 2.750000000000000000 ) ;
#4805=CARTESIAN_POINT ( 'NONE',  ( 2.557341765624996821, -29.71354166700806232, 4.429445870380401828 ) ) ;
#4806=CARTESIAN_POINT ( 'NONE',  ( 2.557341765624996821, -28.71354166700806587, 4.429445870380401828 ) ) ;
#4809=CARTESIAN_POINT ( 'NONE',  ( 6.972266317189433020E-16, -28.68749999999999645, -5.250000000000000000 ) ) ;
#4810=AXIS2_PLACEMENT_3D ( 'NONE', #308, #1006, #7238 ) ;
#4811=DIRECTION ( 'NONE',  ( 0.000000000000000000, 1.000000000000000000, 0.000000000000000000 ) ) ;
#4815=EDGE_CURVE ( 'NONE', #7322, #5643, #3101, .T. ) ;
#4817=CARTESIAN_POINT ( 'NONE',  ( 5.204748896376250699E-16, -30.00000000000000000, -4.250000000000000000 ) ) ;
#4818=CARTESIAN_POINT ( 'NONE',  ( 2.557341765625000818, -29.81770833367473372, -4.429445870380400052 ) ) ;
#4820=VERTEX_POINT ( 'NONE', #5784 ) ;
#4823=CARTESIAN_POINT ( 'NONE',  ( 2.033577675846918216E-14, -27.31250000000000355, 5.250000000000000888 ) ) ;
#4824=CARTESIAN_POINT ( 'NONE',  ( 0.000000000000000000, -9.999999999999998224, 2.750000000000000000 ) ) ;
#4826=CARTESIAN_POINT ( 'NONE',  ( 2.557341765625000818, -28.81770833367473017, -4.429445870380400052 ) ) ;
#4834=CARTESIAN_POINT ( 'NONE',  ( -5.250000000000000000, -27.15625000068279604, -6.429395695523604153E-16 ) ) ;
#4836=EDGE_CURVE ( 'NONE', #1200, #4378, #810, .T. ) ;
#4839=CARTESIAN_POINT ( 'NONE',  ( 2.557341765625000818, -27.31770833367473017, -4.429445870380400052 ) ) ;
#4841=CARTESIAN_POINT ( 'NONE',  ( -5.114683531249999859, -27.31770833367473017, -2.952963913586935440 ) ) ;
#4843=( BOUNDED_CURVE ( )  B_SPLINE_CURVE ( 2, ( #4809, #5461, #6814, #7561, #2543, #6764, #4676, #1142, #440 ),
 .UNSPECIFIED., .F., .T. ) 
 B_SPLINE_CURVE_WITH_KNOTS ( ( 3, 2, 2, 2, 3 ),
 ( 0.4375000000000000000, 0.4444444444444444198, 0.4583333333333333148, 0.4722222222222222099, 0.4791666666666666852 ),
 .UNSPECIFIED. ) 
 CURVE ( )  GEOMETRIC_REPRESENTATION_ITEM ( )  RATIONAL_B_SPLINE_CURVE ( ( 0.9330127018922194093, 0.9330127018922194093, 1.000000000000000000, 0.8660254037844387076, 1.000000000000000000, 0.8660254037844387076, 1.000000000000000000, 0.9330127018922190762, 0.9330127018922194093 ) ) 
 REPRESENTATION_ITEM ( '' )  );
#4844=CARTESIAN_POINT ( 'NONE',  ( -5.114683531250000748, -29.31770833367473017, -2.952963913586935440 ) ) ;
#4846=CARTESIAN_POINT ( 'NONE',  ( 5.114683531249999859, -28.90104166700806942, -2.952963913586932776 ) ) ;
#4855=CARTESIAN_POINT ( 'NONE',  ( 5.114683531249999859, -29.58854166700806232, -2.952963913586932776 ) ) ;
#4864=CARTESIAN_POINT ( 'NONE',  ( 2.625000000000000444, -27.73958333401612819, -4.546633369868303021 ) ) ;
#4865=CARTESIAN_POINT ( 'NONE',  ( -5.114683531250000748, -27.98437500034139802, -6.263680815196995234E-16 ) ) ;
#4869=CARTESIAN_POINT ( 'NONE',  ( -1.975475456537005874E-15, -29.09375000068278894, 5.250000000000000000 ) ) ;
#4872=CARTESIAN_POINT ( 'NONE',  ( 2.300847884672513123E-14, -28.21875000068279604, -5.250000000000000000 ) ) ;
#4875=CARTESIAN_POINT ( 'NONE',  ( 1.185285273922203525E-14, -29.18749999999999645, -5.249999999999999112 ) ) ;
#4876=CARTESIAN_POINT ( 'NONE',  ( 1.406733260263402174, -27.30133545031537068, 5.249999999999995559 ) ) ;
#4881=CARTESIAN_POINT ( 'NONE',  ( 5.114683531250000748, -27.10937500034139802, 0.000000000000000000 ) ) ;
#4883=CARTESIAN_POINT ( 'NONE',  ( -2.557341765625002594, -27.50520833367473017, 4.429445870380399164 ) ) ;
#4885=CARTESIAN_POINT ( 'NONE',  ( -5.114683531250000748, -29.81770833367473372, -2.952963913586935440 ) ) ;
#4888=CARTESIAN_POINT ( 'NONE',  ( 5.114683531249999859, -28.65104166700806587, -2.952963913586932776 ) ) ;
#4890=CARTESIAN_POINT ( 'NONE',  ( 3.367778697655221012E-16, -9.000000000000000000, -2.750000000000000000 ) ) ;
#4893=CARTESIAN_POINT ( 'NONE',  ( 5.249999999999997335, -28.52083333333333215, 3.031088913245538308 ) ) ;
#4898=AXIS2_PLACEMENT_3D ( 'NONE', #84, #6495, #8642 ) ;
#4899=CARTESIAN_POINT ( 'NONE',  ( -2.625000000000002220, -26.86458333401613174, 4.546633369868302132 ) ) ;
#4904=DIRECTION ( 'NONE',  ( 0.000000000000000000, 1.000000000000000000, 0.000000000000000000 ) ) ;
#4907=EDGE_CURVE ( 'NONE', #8178, #5951, #8363, .T. ) ;
#4910=CARTESIAN_POINT ( 'NONE',  ( 5.250000000000000000, -27.78125000068279604, 0.000000000000000000 ) ) ;
#4912=CARTESIAN_POINT ( 'NONE',  ( 2.557341765624996821, -29.15104166700806587, 4.429445870380401828 ) ) ;
#4920=CARTESIAN_POINT ( 'NONE',  ( 0.000000000000000000, -9.999999999999998224, 0.000000000000000000 ) ) ;
#4924=CARTESIAN_POINT ( 'NONE',  ( -2.557341765624999042, -27.27604166700806587, -4.429445870380400052 ) ) ;
#4926=CARTESIAN_POINT ( 'NONE',  ( 2.625000000000000444, -28.70833333333333215, -4.546633369868303021 ) ) ;
#4927=CARTESIAN_POINT ( 'NONE',  ( 0.000000000000000000, -30.00000000000000000, 0.000000000000000000 ) ) ;
#4928=EDGE_CURVE ( 'NONE', #6454, #8645, #4843, .T. ) ;
#4929=CARTESIAN_POINT ( 'NONE',  ( 5.114683531249998971, -29.19270833367473017, 2.952963913586936329 ) ) ;
#4931=CARTESIAN_POINT ( 'NONE',  ( 5.114683531249999859, -27.15104166700806232, -2.952963913586932776 ) ) ;
#4932=CARTESIAN_POINT ( 'NONE',  ( -5.250000000000000888, -28.38541666734946389, 3.031088913245533423 ) ) ;
#4935=AXIS2_PLACEMENT_3D ( 'NONE', #4132, #2506, #405 ) ;
#4941=CARTESIAN_POINT ( 'NONE',  ( -1.084901341431563923E-15, -29.17187500034139802, 5.905927827173866440 ) ) ;
#4942=ADVANCED_FACE ( 'NONE', ( #1187, #4031 ), #6165, .F. ) ;
#4947=DIRECTION ( 'NONE',  ( 0.000000000000000000, 1.000000000000000000, 0.000000000000000000 ) ) ;
#4949=CARTESIAN_POINT ( 'NONE',  ( -2.625000000000002220, -27.58333333333333215, 4.546633369868302132 ) ) ;
#4952=CARTESIAN_POINT ( 'NONE',  ( 5.114683531249998971, -29.13020833367473372, 2.952963913586936329 ) ) ;
#4955=CARTESIAN_POINT ( 'NONE',  ( -1.975475456537005874E-15, -28.84375000068279959, 5.250000000000000000 ) ) ;
#4963=VERTEX_POINT ( 'NONE', #2774 ) ;
#4967=DIRECTION ( 'NONE',  ( 0.000000000000000000, 1.000000000000000000, 0.000000000000000000 ) ) ;
#4970=CARTESIAN_POINT ( 'NONE',  ( 2.625000000000000444, -29.45833333333333215, -4.546633369868303021 ) ) ;
#4971=EDGE_CURVE ( 'NONE', #874, #8929, #4163, .T. ) ;
#4972=CARTESIAN_POINT ( 'NONE',  ( -5.114683531250001636, -29.77604166700806232, 2.952963913586931444 ) ) ;
#4973=CARTESIAN_POINT ( 'NONE',  ( -5.114683531250000748, -28.27604166700806232, 2.952963913586931888 ) ) ;
#4975=CYLINDRICAL_SURFACE ( 'NONE', #7776, 5.250000000000000000 ) ;
#4977=CARTESIAN_POINT ( 'NONE',  ( 5.182341765625000818, -29.96093750017069723, 0.000000000000000000 ) ) ;
#4980=ORIENTED_EDGE ( 'NONE', *, *, #4815, .F. ) ;
#4982=CARTESIAN_POINT ( 'NONE',  ( 5.114683531249998971, -29.63020833367473017, 2.952963913586936329 ) ) ;
#4983=ORIENTED_EDGE ( 'NONE', *, *, #3446, .F. ) ;
#4984=ORIENTED_EDGE ( 'NONE', *, *, #7742, .T. ) ;
#4987=CARTESIAN_POINT ( 'NONE',  ( 0.000000000000000000, -30.00000000000000000, 5.250000000000000000 ) ) ;
#4988=EDGE_LOOP ( 'NONE', ( #111, #8103, #4536, #6582 ) ) ;
#4993=CARTESIAN_POINT ( 'NONE',  ( 5.114683531249998971, -28.13020833367473017, 2.952963913586936329 ) ) ;
#5002=CARTESIAN_POINT ( 'NONE',  ( -5.250000000000000888, -27.63541666734946389, 3.031088913245533423 ) ) ;
#5011=CARTESIAN_POINT ( 'NONE',  ( 2.624999999999996891, -28.79166666666666785, 4.546633369868304797 ) ) ;
#5012=FACE_OUTER_BOUND ( 'NONE', #7500, .T. ) ;
#5014=CARTESIAN_POINT ( 'NONE',  ( 5.114683531249998971, -27.44270833367472662, 2.952963913586936329 ) ) ;
#5015=CIRCLE ( 'NONE', #1024, 5.250000000000000000 ) ;
#5017=CARTESIAN_POINT ( 'NONE',  ( 2.557341765625000818, -28.13020833367473017, -4.429445870380400052 ) ) ;
#5018=FACE_OUTER_BOUND ( 'NONE', #8154, .T. ) ;
#5028=CARTESIAN_POINT ( 'NONE',  ( -5.114683531249999859, -28.75520833367473017, -2.952963913586935440 ) ) ;
#5029=VERTEX_POINT ( 'NONE', #4205 ) ;
#5030=ORIENTED_EDGE ( 'NONE', *, *, #6824, .T. ) ;
#5031=CIRCLE ( 'NONE', #3269, 2.750000000000000000 ) ;
#5039=CARTESIAN_POINT ( 'NONE',  ( -5.249999999999999112, -27.64583333333333215, -3.031088913245536975 ) ) ;
#5042=CARTESIAN_POINT ( 'NONE',  ( 1.406733260263402174, -27.83258545099816672, 5.249999999999995559 ) ) ;
#5043=CARTESIAN_POINT ( 'NONE',  ( -5.114683531250000748, -27.23437500034139802, -6.263680815196995234E-16 ) ) ;
#5054=CARTESIAN_POINT ( 'NONE',  ( 0.000000000000000000, -9.000000000000000000, 0.000000000000000000 ) ) ;
#5057=ORIENTED_EDGE ( 'NONE', *, *, #6326, .T. ) ;
#5061=CARTESIAN_POINT ( 'NONE',  ( -5.250000000000000888, -29.60416666666666430, 3.031088913245532979 ) ) ;
#5062=CARTESIAN_POINT ( 'NONE',  ( 5.204748896376250699E-16, 75.00000000000000000, -4.250000000000000000 ) ) ;
#5063=CARTESIAN_POINT ( 'NONE',  ( 5.114683531250000748, -27.90104166700806587, -2.952963913586932776 ) ) ;
#5064=CARTESIAN_POINT ( 'NONE',  ( 5.114683531250000748, -27.42187500034139802, 0.000000000000000000 ) ) ;
#5065=CARTESIAN_POINT ( 'NONE',  ( 3.616337804771879580E-16, -29.79687500034139447, -5.905927827173866440 ) ) ;
#5068=ADVANCED_FACE ( 'NONE', ( #7830 ), #4975, .T. ) ;
#5071=CARTESIAN_POINT ( 'NONE',  ( -5.114683531250000748, -29.54687500034139802, -6.263680815196995234E-16 ) ) ;
#5076=CARTESIAN_POINT ( 'NONE',  ( -2.557341765625002594, -28.69270833367473017, 4.429445870380399164 ) ) ;
#5077=( BOUNDED_CURVE ( )  B_SPLINE_CURVE ( 2, ( #1788, #382, #8109, #5356, #4574, #8204, #6802, #7550, #8934 ),
 .UNSPECIFIED., .F., .T. ) 
 B_SPLINE_CURVE_WITH_KNOTS ( ( 3, 2, 2, 2, 3 ),
 ( 0.6041666666666666297, 0.6111111111111111605, 0.6250000000000000000, 0.6388888888888888395, 0.6458333333333333703 ),
 .UNSPECIFIED. ) 
 CURVE ( )  GEOMETRIC_REPRESENTATION_ITEM ( )  RATIONAL_B_SPLINE_CURVE ( ( 0.9330127018922192983, 0.9330127018922187432, 1.000000000000000000, 0.8660254037844387076, 1.000000000000000000, 0.8660254037844387076, 1.000000000000000000, 0.9330127018922187432, 0.9330127018922192983 ) ) 
 REPRESENTATION_ITEM ( '' )  );
#5081=EDGE_CURVE ( 'NONE', #1056, #8090, #7028, .T. ) ;
#5090=CARTESIAN_POINT ( 'NONE',  ( 5.250000000000000000, -29.53125000068279604, 0.000000000000000000 ) ) ;
#5092=AXIS2_PLACEMENT_3D ( 'NONE', #7876, #1495, #6465 ) ;
#5093=CARTESIAN_POINT ( 'NONE',  ( -5.114683531250000748, -26.98437500034139802, -6.263680815196995234E-16 ) ) ;
#5100=DIRECTION ( 'NONE',  ( 0.000000000000000000, 1.000000000000000000, 0.000000000000000000 ) ) ;
#5103=VERTEX_POINT ( 'NONE', #798 ) ;
#5106=LINE ( 'NONE', #1317, #5764 ) ;
#5111=CARTESIAN_POINT ( 'NONE',  ( -5.250000000000000000, -29.14583333333333925, -3.031088913245536531 ) ) ;
#5113=CARTESIAN_POINT ( 'NONE',  ( -5.114683531250001636, -27.27604166700806587, 2.952963913586931444 ) ) ;
#5116=LINE ( 'NONE', #7963, #4645 ) ;
#5119=CARTESIAN_POINT ( 'NONE',  ( 1.406733260263397289, -28.80133545031537423, 5.249999999999997335 ) ) ;
#5120=CARTESIAN_POINT ( 'NONE',  ( -5.114683531249999859, -29.81770833367473017, -2.952963913586935440 ) ) ;
#5121=CARTESIAN_POINT ( 'NONE',  ( 2.624999999999996891, -28.32291666734946389, 4.546633369868304797 ) ) ;
#5124=CARTESIAN_POINT ( 'NONE',  ( 2.033577675846918216E-14, -28.06249999999999645, 5.250000000000000888 ) ) ;
#5125=CARTESIAN_POINT ( 'NONE',  ( -2.557341765625002594, -28.44270833367473017, 4.429445870380399164 ) ) ;
#5135=ADVANCED_FACE ( 'NONE', ( #7969 ), #7925, .F. ) ;
#5137=CARTESIAN_POINT ( 'NONE',  ( -2.625000000000002220, -29.36458333401613174, 4.546633369868302132 ) ) ;
#5139=CARTESIAN_POINT ( 'NONE',  ( -2.557341765624999042, -29.83854166700806232, -4.429445870380400052 ) ) ;
#5158=EDGE_CURVE ( 'NONE', #3172, #3585, #3308, .T. ) ;
#5161=CARTESIAN_POINT ( 'NONE',  ( -5.250000000000000000, -27.37500000000000000, -6.429395695523604153E-16 ) ) ;
#5163=CARTESIAN_POINT ( 'NONE',  ( -2.557341765624999042, -27.83854166700806587, -4.429445870380400052 ) ) ;
#5166=CARTESIAN_POINT ( 'NONE',  ( 0.000000000000000000, -30.00000000000000000, 5.250000000000000000 ) ) ;
#5169=CARTESIAN_POINT ( 'NONE',  ( -5.250000000000000000, -27.40625000068279604, -6.429395695523604153E-16 ) ) ;
#5170=CARTESIAN_POINT ( 'NONE',  ( -5.114683531249999859, -29.06770833367473017, -2.952963913586935440 ) ) ;
#5171=CARTESIAN_POINT ( 'NONE',  ( 5.250000000000000000, -28.28125000068279604, 0.000000000000000000 ) ) ;
#5175=CARTESIAN_POINT ( 'NONE',  ( 2.557341765625000818, -27.81770833367473017, -4.429445870380400052 ) ) ;
#5176=AXIS2_PLACEMENT_3D ( 'NONE', #3728, #5204, #4606 ) ;
#5178=CARTESIAN_POINT ( 'NONE',  ( 1.406733260263402174, -26.83258545099816672, 5.249999999999995559 ) ) ;
#5184=CARTESIAN_POINT ( 'NONE',  ( 6.972266317189433020E-16, -29.71875000068279249, -5.249999999999999112 ) ) ;
#5185=CARTESIAN_POINT ( 'NONE',  ( 5.250000000000000000, -29.01041666734946389, -3.031088913245534755 ) ) ;
#5188=CARTESIAN_POINT ( 'NONE',  ( -1.084901341431563923E-15, -29.73437500034140157, 5.905927827173866440 ) ) ;
#5189=ORIENTED_EDGE ( 'NONE', *, *, #609, .T. ) ;
#5193=CARTESIAN_POINT ( 'NONE',  ( 0.000000000000000000, -30.00000000000000000, 0.000000000000000000 ) ) ;
#5204=DIRECTION ( 'NONE',  ( 0.000000000000000000, 1.000000000000000000, 0.000000000000000000 ) ) ;
#5210=CARTESIAN_POINT ( 'NONE',  ( 5.249999999999999112, -28.27083333333332860, 3.031088913245538308 ) ) ;
#5211=CARTESIAN_POINT ( 'NONE',  ( 2.557341765625000818, -27.88020833367473017, -4.429445870380400052 ) ) ;
#5212=PRESENTATION_STYLE_ASSIGNMENT (( #6749 ) ) ;
#5213=CARTESIAN_POINT ( 'NONE',  ( -5.250000000000000888, -29.38541666734946034, 3.031088913245533423 ) ) ;
#5217=CARTESIAN_POINT ( 'NONE',  ( 5.250000000000000000, -28.78125000068279604, 0.000000000000000000 ) ) ;
#5218=LINE ( 'NONE', #287, #494 ) ;
#5219=CARTESIAN_POINT ( 'NONE',  ( -2.557341765624999042, -28.83854166700806587, -4.429445870380400052 ) ) ;
#5221=VERTEX_POINT ( 'NONE', #6659 ) ;
#5223=CARTESIAN_POINT ( 'NONE',  ( 2.557341765625000818, -29.06770833367473017, -4.429445870380400052 ) ) ;
#5224=EDGE_LOOP ( 'NONE', ( #7973, #714, #2421, #3677, #8977, #710 ) ) ;
#5231=CARTESIAN_POINT ( 'NONE',  ( -5.250000000000000000, -29.87500000000000000, -6.429395695523604153E-16 ) ) ;
#5232=CARTESIAN_POINT ( 'NONE',  ( 5.250000000000000000, -28.78125000068279604, 0.000000000000000000 ) ) ;
#5233=EDGE_CURVE ( 'NONE', #5696, #4680, #331, .T. ) ;
#5235=CARTESIAN_POINT ( 'NONE',  ( 3.616337804771879580E-16, -27.04687500034139802, -5.905927827173866440 ) ) ;
#5236=EDGE_LOOP ( 'NONE', ( #8105, #4578, #5814, #832 ) ) ;
#5239=LINE ( 'NONE', #5285, #1325 ) ;
#5255=CARTESIAN_POINT ( 'NONE',  ( -1.113604000661152470E-15, -28.31250000000000000, 6.062177826491070398 ) ) ;
#5257=EDGE_LOOP ( 'NONE', ( #91, #988, #7364, #1826 ) ) ;
#5259=VERTEX_POINT ( 'NONE', #8206 ) ;
#5261=CARTESIAN_POINT ( 'NONE',  ( -5.114683531250001636, -28.46354166700806587, 2.952963913586931444 ) ) ;
#5265=CARTESIAN_POINT ( 'NONE',  ( 5.114683531250000748, -28.92187500034139802, 0.000000000000000000 ) ) ;
#5268=CARTESIAN_POINT ( 'NONE',  ( -1.975475456537005874E-15, -29.31250000000000000, 5.250000000000000000 ) ) ;
#5269=CARTESIAN_POINT ( 'NONE',  ( 5.114683531249998971, -27.13020833367473372, 2.952963913586936329 ) ) ;
#5270=APPLICATION_CONTEXT ( 'automotive_design' ) ;
#5271=EDGE_LOOP ( 'NONE', ( #5362, #8247, #1897, #8896 ) ) ;
#5272=( BOUNDED_CURVE ( )  B_SPLINE_CURVE ( 2, ( #3616, #5042, #1424, #8634, #4910, #6441, #4864, #680, #638 ),
 .UNSPECIFIED., .F., .T. ) 
 B_SPLINE_CURVE_WITH_KNOTS ( ( 3, 2, 2, 2, 3 ),
 ( 0.6458333333333333703, 0.6527777777777777901, 0.6666666666666666297, 0.6805555555555555802, 0.6875000000000000000 ),
 .UNSPECIFIED. ) 
 CURVE ( )  GEOMETRIC_REPRESENTATION_ITEM ( )  RATIONAL_B_SPLINE_CURVE ( ( 0.9330127018922192983, 0.9330127018922198534, 1.000000000000000000, 0.8660254037844387076, 1.000000000000000000, 0.8660254037844387076, 1.000000000000000000, 0.9330127018922194093, 0.9330127018922194093 ) ) 
 REPRESENTATION_ITEM ( '' )  );
#5276=CARTESIAN_POINT ( 'NONE',  ( 1.185285273922203525E-14, -29.18750000000000000, -5.250000000000000000 ) ) ;
#5280=CARTESIAN_POINT ( 'NONE',  ( -5.250000000000000000, -29.67708333401613174, -3.031088913245536531 ) ) ;
#5285=CARTESIAN_POINT ( 'NONE',  ( 0.000000000000000000, -30.00000000000000000, 5.250000000000000000 ) ) ;
#5293=CARTESIAN_POINT ( 'NONE',  ( -2.625000000000002220, -29.58333333333333215, 4.546633369868302132 ) ) ;
#5294=ORIENTED_EDGE ( 'NONE', *, *, #3331, .F. ) ;
#5298=CARTESIAN_POINT ( 'NONE',  ( -2.625000000000002220, -28.08333333333333215, 4.546633369868302132 ) ) ;
#5301=ORIENTED_EDGE ( 'NONE', *, *, #7310, .F. ) ;
#5304=CARTESIAN_POINT ( 'NONE',  ( -1.084901341431563726E-15, -28.42187500034139802, 5.905927827173866440 ) ) ;
#5307=CARTESIAN_POINT ( 'NONE',  ( 2.624999999999996891, -28.57291666734946389, 4.546633369868304797 ) ) ;
#5308=CARTESIAN_POINT ( 'NONE',  ( 5.114683531249999859, -28.15104166700806587, -2.952963913586932776 ) ) ;
#5309=CARTESIAN_POINT ( 'NONE',  ( 5.249999999999999112, -27.26041666734946034, -3.031088913245534755 ) ) ;
#5312=CARTESIAN_POINT ( 'NONE',  ( 5.114683531249998971, -27.38020833367473017, 2.952963913586936329 ) ) ;
#5316=CYLINDRICAL_SURFACE ( 'NONE', #3709, 5.250000000000000000 ) ;
#5321=FACE_OUTER_BOUND ( 'NONE', #2376, .T. ) ;
#5322=CARTESIAN_POINT ( 'NONE',  ( 3.712013335537174572E-16, -27.96875000068279604, -6.062177826491070398 ) ) ;
#5324=EDGE_LOOP ( 'NONE', ( #2323, #4490 ) ) ;
#5325=CIRCLE ( 'NONE', #1933, 4.250000000000000000 ) ;
#5328=CARTESIAN_POINT ( 'NONE',  ( 2.625000000000000444, -29.45833333333333215, -4.546633369868303021 ) ) ;
#5331=ADVANCED_FACE ( 'NONE', ( #7603 ), #4713, .T. ) ;
#5332=CARTESIAN_POINT ( 'NONE',  ( 0.000000000000000000, -9.000000000000000000, 0.000000000000000000 ) ) ;
#5336=DIRECTION ( 'NONE',  ( 0.000000000000000000, 1.000000000000000000, 0.000000000000000000 ) ) ;
#5337=CARTESIAN_POINT ( 'NONE',  ( 2.033577675846918216E-14, -27.81249999999999645, 5.250000000000000888 ) ) ;
#5341=CARTESIAN_POINT ( 'NONE',  ( -1.975475456537005874E-15, -29.56250000000000000, 5.250000000000000000 ) ) ;
#5345=CARTESIAN_POINT ( 'NONE',  ( 2.625000000000000444, -28.20833333333333215, -4.546633369868303021 ) ) ;
#5348=CARTESIAN_POINT ( 'NONE',  ( 3.616337804771879580E-16, -27.10937500034139802, -5.905927827173866440 ) ) ;
#5351=AXIS2_PLACEMENT_3D ( 'NONE', #8337, #9021, #6146 ) ;
#5352=ORIENTED_EDGE ( 'NONE', *, *, #4928, .F. ) ;
#5353=CARTESIAN_POINT ( 'NONE',  ( 3.616337804771879580E-16, -29.04687500034139802, -5.905927827173866440 ) ) ;
#5356=CARTESIAN_POINT ( 'NONE',  ( -5.249999999999999112, -28.14583333333333215, -3.031088913245536975 ) ) ;
#5357=CARTESIAN_POINT ( 'NONE',  ( 2.557341765625000818, -28.63020833367473017, -4.429445870380400052 ) ) ;
#5360=AXIS2_PLACEMENT_3D ( 'NONE', #3244, #447, #4725 ) ;
#5361=CARTESIAN_POINT ( 'NONE',  ( 5.114683531249998971, -26.88020833367473017, 2.952963913586936329 ) ) ;
#5362=ORIENTED_EDGE ( 'NONE', *, *, #191, .F. ) ;
#5363=EDGE_CURVE ( 'NONE', #8492, #6529, #8225, .T. ) ;
#5372=CARTESIAN_POINT ( 'NONE',  ( 5.250000000000000000, -28.26041666734946745, -3.031088913245534755 ) ) ;
#5380=DIRECTION ( 'NONE',  ( 0.000000000000000000, 0.000000000000000000, 1.000000000000000000 ) ) ;
#5383=CARTESIAN_POINT ( 'NONE',  ( 5.114683531250000748, -29.35937500034139802, 0.000000000000000000 ) ) ;
#5395=VECTOR ( 'NONE', #6893, 1000.000000000000000 ) ;
#5396=CIRCLE ( 'NONE', #8820, 5.250000000000000000 ) ;
#5400=ORIENTED_EDGE ( 'NONE', *, *, #8283, .T. ) ;
#5401=CARTESIAN_POINT ( 'NONE',  ( 2.557341765624996821, -28.90104166700806587, 4.429445870380401828 ) ) ;
#5403=DIRECTION ( 'NONE',  ( 0.000000000000000000, 0.000000000000000000, 1.000000000000000000 ) ) ;
#5404=CARTESIAN_POINT ( 'NONE',  ( 2.557341765625000818, -27.13020833367473017, -4.429445870380400052 ) ) ;
#5406=CARTESIAN_POINT ( 'NONE',  ( 0.000000000000000000, -9.000000000000000000, 2.750000000000000000 ) ) ;
#5407=CARTESIAN_POINT ( 'NONE',  ( 2.557341765624996821, -27.15104166700806587, 4.429445870380401828 ) ) ;
#5409=CARTESIAN_POINT ( 'NONE',  ( -5.250000000000000888, -28.35416666666666785, 3.031088913245533423 ) ) ;
#5410=CARTESIAN_POINT ( 'NONE',  ( 2.557341765624996821, -28.96354166700806587, 4.429445870380401828 ) ) ;
#5419=CARTESIAN_POINT ( 'NONE',  ( 5.250000000000000000, -27.51041666734946389, -3.031088913245534755 ) ) ;
#5428=LINE ( 'NONE', #3952, #8809 ) ;
#5442=( BOUNDED_CURVE ( )  B_SPLINE_CURVE ( 2, ( #9130, #3465, #7130, #752, #9086, #8355, #6254, #2110, #1320 ),
 .UNSPECIFIED., .F., .F. ) 
 B_SPLINE_CURVE_WITH_KNOTS ( ( 3, 2, 2, 2, 3 ),
 ( 0.06250000000000000000, 0.06944444444444444753, 0.08333333333333332871, 0.09722222222222222376, 0.1041666666666666713 ),
 .UNSPECIFIED. ) 
 CURVE ( )  GEOMETRIC_REPRESENTATION_ITEM ( )  RATIONAL_B_SPLINE_CURVE ( ( 0.9330127018922194093, 0.9330127018922194093, 1.000000000000000000, 0.8660254037844387076, 1.000000000000000000, 0.8660254037844387076, 1.000000000000000000, 0.9330127018922192983, 0.9330127018922194093 ) ) 
 REPRESENTATION_ITEM ( '' )  );
#5447=ORIENTED_EDGE ( 'NONE', *, *, #8719, .T. ) ;
#5449=CARTESIAN_POINT ( 'NONE',  ( -2.557341765624999042, -28.77604166700806587, -4.429445870380400052 ) ) ;
#5452=CARTESIAN_POINT ( 'NONE',  ( 3.616337804771879580E-16, -27.10937500034139802, -5.905927827173866440 ) ) ;
#5455=CARTESIAN_POINT ( 'NONE',  ( -5.114683531249999859, -27.00520833367473017, -2.952963913586935440 ) ) ;
#5457=CARTESIAN_POINT ( 'NONE',  ( 3.616337804771879580E-16, -28.60937500034139802, -5.905927827173866440 ) ) ;
#5461=CARTESIAN_POINT ( 'NONE',  ( -1.406733260263393293, -28.67633545031537068, -5.250000000000000000 ) ) ;
#5465=ORIENTED_EDGE ( 'NONE', *, *, #4971, .F. ) ;
#5467=CARTESIAN_POINT ( 'NONE',  ( -5.250000000000000888, -27.63541666734946034, 3.031088913245532979 ) ) ;
#5473=CARTESIAN_POINT ( 'NONE',  ( 6.972266317189433020E-16, -29.71875000068279249, -5.250000000000000000 ) ) ;
#5478=CARTESIAN_POINT ( 'NONE',  ( 5.114683531249999859, -29.83854166700806587, -2.952963913586932776 ) ) ;
#5487=CARTESIAN_POINT ( 'NONE',  ( -5.249999999999999112, -27.17708333401612819, -3.031088913245536975 ) ) ;
#5491=EDGE_LOOP ( 'NONE', ( #5301, #2230, #6170, #353 ) ) ;
#5496=ADVANCED_FACE ( 'NONE', ( #2190 ), #4153, .F. ) ;
#5497=CARTESIAN_POINT ( 'NONE',  ( 5.114683531250000748, -27.58854166700806587, -2.952963913586932776 ) ) ;
#5501=CARTESIAN_POINT ( 'NONE',  ( 5.250000000000000000, -29.97916666666666430, -3.031088913245534755 ) ) ;
#5502=DIRECTION ( 'NONE',  ( 1.000000000000000000, 0.000000000000000000, 0.000000000000000000 ) ) ;
#5504=( BOUNDED_CURVE ( )  B_SPLINE_CURVE ( 2, ( #4869, #7810, #5614, #1344, #4268, #8462, #775, #3575, #5748 ),
 .UNSPECIFIED., .F., .F. ) 
 B_SPLINE_CURVE_WITH_KNOTS ( ( 3, 2, 2, 2, 3 ),
 ( 0.2291666666666666574, 0.2361111111111111049, 0.2500000000000000000, 0.2638888888888888951, 0.2708333333333333148 ),
 .UNSPECIFIED. ) 
 CURVE ( )  GEOMETRIC_REPRESENTATION_ITEM ( )  RATIONAL_B_SPLINE_CURVE ( ( 0.9330127018922194093, 0.9330127018922194093, 1.000000000000000000, 0.8660254037844387076, 1.000000000000000000, 0.8660254037844387076, 1.000000000000000000, 0.9330127018922196314, 0.9330127018922194093 ) ) 
 REPRESENTATION_ITEM ( '' )  );
#5505=CARTESIAN_POINT ( 'NONE',  ( 2.557341765625000818, -28.88020833367473017, -4.429445870380400052 ) ) ;
#5508=CARTESIAN_POINT ( 'NONE',  ( -5.114683531250000748, -28.79687500034139802, -6.263680815196995234E-16 ) ) ;
#5511=CARTESIAN_POINT ( 'NONE',  ( -2.624999999999998668, -29.19791666734946389, -4.546633369868303021 ) ) ;
#5516=ORIENTED_EDGE ( 'NONE', *, *, #6725, .F. ) ;
#5517=CARTESIAN_POINT ( 'NONE',  ( 2.033577675846918216E-14, -27.81249999999999645, 5.250000000000000888 ) ) ;
#5518=CARTESIAN_POINT ( 'NONE',  ( 3.712013335537174572E-16, -28.46875000068279249, -6.062177826491070398 ) ) ;
#5523=CYLINDRICAL_SURFACE ( 'NONE', #9186, 5.250000000000000000 ) ;
#5524=( BOUNDED_CURVE ( )  B_SPLINE_CURVE ( 2, ( #1412, #7968, #8664, #7833, #3002, #1499, #5684, #7132, #4252 ),
 .UNSPECIFIED., .F., .T. ) 
 B_SPLINE_CURVE_WITH_KNOTS ( ( 3, 2, 2, 2, 3 ),
 ( 0.02083333333333333218, 0.02777777777777777624, 0.04166666666666666435, 0.05555555555555555247, 0.06250000000000000000 ),
 .UNSPECIFIED. ) 
 CURVE ( )  GEOMETRIC_REPRESENTATION_ITEM ( )  RATIONAL_B_SPLINE_CURVE ( ( 0.9330127018922194093, 0.9330127018922194093, 1.000000000000000000, 0.8660254037844387076, 1.000000000000000000, 0.8660254037844387076, 1.000000000000000000, 0.9330127018922194093, 0.9330127018922194093 ) ) 
 REPRESENTATION_ITEM ( '' )  );
#5529=CARTESIAN_POINT ( 'NONE',  ( -5.114683531250000748, -28.23437500034139447, -6.263680815196995234E-16 ) ) ;
#5539=ORIENTED_EDGE ( 'NONE', *, *, #7576, .T. ) ;
#5542=CARTESIAN_POINT ( 'NONE',  ( -5.114683531250000748, -27.73437500034139802, -6.263680815196995234E-16 ) ) ;
#5544=CARTESIAN_POINT ( 'NONE',  ( -5.114683531250000748, -27.29687500034139802, -6.263680815196995234E-16 ) ) ;
#5547=CARTESIAN_POINT ( 'NONE',  ( -1.084901341431563726E-15, -29.48437500034139802, 5.905927827173866440 ) ) ;
#5548=EDGE_CURVE ( 'NONE', #4820, #4350, #793, .T. ) ;
#5549=CARTESIAN_POINT ( 'NONE',  ( 2.557341765625000818, -29.63020833367473017, -4.429445870380400052 ) ) ;
#5555=CARTESIAN_POINT ( 'NONE',  ( 5.250000000000000000, -28.49999999999999645, 0.000000000000000000 ) ) ;
#5560=CARTESIAN_POINT ( 'NONE',  ( 2.625000000000000444, -27.23958333401612819, -4.546633369868303021 ) ) ;
#5565=CARTESIAN_POINT ( 'NONE',  ( -5.250000000000000888, -27.10416666666666430, 3.031088913245533423 ) ) ;
#5570=CARTESIAN_POINT ( 'NONE',  ( 5.114683531250000748, -28.85937500034139802, 0.000000000000000000 ) ) ;
#5572=CARTESIAN_POINT ( 'NONE',  ( -1.975475456537005874E-15, -29.09375000068279249, 5.249999999999999112 ) ) ;
#5574=CARTESIAN_POINT ( 'NONE',  ( 0.000000000000000000, -9.999999999999998224, 0.000000000000000000 ) ) ;
#5578=CARTESIAN_POINT ( 'NONE',  ( 6.972266317189433020E-16, -27.71875000068279604, -5.249999999999999112 ) ) ;
#5584=CARTESIAN_POINT ( 'NONE',  ( -2.557341765624999042, -28.02604166700806587, -4.429445870380400052 ) ) ;
#5586=CARTESIAN_POINT ( 'NONE',  ( -1.084901341431563923E-15, -27.48437500034140157, 5.905927827173866440 ) ) ;
#5589=CARTESIAN_POINT ( 'NONE',  ( 2.557341765625000818, -29.63020833367473017, -4.429445870380400052 ) ) ;
#5591=CARTESIAN_POINT ( 'NONE',  ( -2.557341765625002594, -29.00520833367473017, 4.429445870380399164 ) ) ;
#5595=ADVANCED_FACE ( 'NONE', ( #5012 ), #93, .T. ) ;
#5601=CARTESIAN_POINT ( 'NONE',  ( -2.624999999999998668, -26.94791666734946389, -4.546633369868303021 ) ) ;
#5606=CARTESIAN_POINT ( 'NONE',  ( -5.250000000000000000, -27.12500000000000000, -6.429395695523604153E-16 ) ) ;
#5607=ORIENTED_EDGE ( 'NONE', *, *, #6672, .F. ) ;
#5612=CARTESIAN_POINT ( 'NONE',  ( 3.616337804771879580E-16, -28.54687500034139802, -5.905927827173866440 ) ) ;
#5614=CARTESIAN_POINT ( 'NONE',  ( 2.624999999999996891, -29.07291666734946389, 4.546633369868304797 ) ) ;
#5620=FACE_BOUND ( 'NONE', #5324, .T. ) ;
#5625=CIRCLE ( 'NONE', #6826, 5.250000000000000000 ) ;
#5627=CARTESIAN_POINT ( 'NONE',  ( 3.616337804771879580E-16, -27.54687500034139802, -5.905927827173866440 ) ) ;
#5629=CARTESIAN_POINT ( 'NONE',  ( -1.113604000661152470E-15, -28.81249999999999645, 6.062177826491070398 ) ) ;
#5631=CARTESIAN_POINT ( 'NONE',  ( -5.114683531250000748, -29.79687500034139802, -6.263680815196995234E-16 ) ) ;
#5634=CARTESIAN_POINT ( 'NONE',  ( -2.557341765625002594, -27.25520833367473017, 4.429445870380399164 ) ) ;
#5643=VERTEX_POINT ( 'NONE', #5062 ) ;
#5646=CARTESIAN_POINT ( 'NONE',  ( -2.557341765625002594, -29.19270833367473017, 4.429445870380399164 ) ) ;
#5648=ORIENTED_EDGE ( 'NONE', *, *, #3349, .F. ) ;
#5655=EDGE_CURVE ( 'NONE', #4378, #1880, #5789, .T. ) ;
#5658=CARTESIAN_POINT ( 'NONE',  ( 5.114683531250000748, -29.10937500034139802, 0.000000000000000000 ) ) ;
#5661=EDGE_CURVE ( 'NONE', #5696, #7888, #6781, .T. ) ;
#5666=FACE_BOUND ( 'NONE', #8123, .T. ) ;
#5667=CARTESIAN_POINT ( 'NONE',  ( -5.249999999999999112, -27.89583333333332860, -3.031088913245536975 ) ) ;
#5668=ORIENTED_EDGE ( 'NONE', *, *, #698, .F. ) ;
#5671=CARTESIAN_POINT ( 'NONE',  ( -2.557341765624999042, -27.77604166700806587, -4.429445870380400052 ) ) ;
#5673=CARTESIAN_POINT ( 'NONE',  ( -5.250000000000000000, -28.89583333333333215, -3.031088913245536531 ) ) ;
#5675=CARTESIAN_POINT ( 'NONE',  ( -2.557341765625002594, -29.50520833367473017, 4.429445870380399164 ) ) ;
#5678=CARTESIAN_POINT ( 'NONE',  ( -5.114683531249999859, -27.31770833367473017, -2.952963913586935440 ) ) ;
#5682=VECTOR ( 'NONE', #3028, 1000.000000000000000 ) ;
#5684=CARTESIAN_POINT ( 'NONE',  ( -2.625000000000002220, -29.61458333401613174, 4.546633369868302132 ) ) ;
#5689=CARTESIAN_POINT ( 'NONE',  ( 5.114683531249999859, -29.33854166700805877, -2.952963913586932776 ) ) ;
#5696=VERTEX_POINT ( 'NONE', #7581 ) ;
#5701=CARTESIAN_POINT ( 'NONE',  ( -5.114683531250000748, -28.73437500034139802, -6.263680815196995234E-16 ) ) ;
#5705=DIRECTION ( 'NONE',  ( 0.000000000000000000, 1.000000000000000000, 0.000000000000000000 ) ) ;
#5708=( LENGTH_UNIT ( ) NAMED_UNIT ( * ) SI_UNIT ( .MILLI., .METRE. ) );
#5710=CARTESIAN_POINT ( 'NONE',  ( -1.406733260263393293, -27.70758545099817027, -5.250000000000000000 ) ) ;
#5714=ORIENTED_EDGE ( 'NONE', *, *, #6059, .T. ) ;
#5718=CARTESIAN_POINT ( 'NONE',  ( 2.625000000000000444, -29.20833333333333215, -4.546633369868303021 ) ) ;
#5720=CARTESIAN_POINT ( 'NONE',  ( -5.114683531250000748, -27.56770833367473017, -2.952963913586935440 ) ) ;
#5721=CARTESIAN_POINT ( 'NONE',  ( -5.114683531250000748, -28.29687500034139447, -6.263680815196995234E-16 ) ) ;
#5723=LINE ( 'NONE', #5166, #5943 ) ;
#5729=ORIENTED_EDGE ( 'NONE', *, *, #2044, .F. ) ;
#5732=CARTESIAN_POINT ( 'NONE',  ( -5.114683531249999859, -28.50520833367473017, -2.952963913586935440 ) ) ;
#5736=CARTESIAN_POINT ( 'NONE',  ( 6.429395695523604153E-16, -30.00000000000000000, -5.250000000000000000 ) ) ;
#5740=CARTESIAN_POINT ( 'NONE',  ( -1.975475456537005874E-15, -27.56249999999999289, 5.250000000000000000 ) ) ;
#5742=STYLED_ITEM ( 'NONE', ( #5212 ), #4641 ) ;
#5745=CARTESIAN_POINT ( 'NONE',  ( 5.114683531249999859, -27.83854166700806587, -2.952963913586932776 ) ) ;
#5748=CARTESIAN_POINT ( 'NONE',  ( 1.185285273922203525E-14, -28.96875000068279959, -5.250000000000000000 ) ) ;
#5750=CARTESIAN_POINT ( 'NONE',  ( -5.250000000000000888, -28.13541666734947100, 3.031088913245533423 ) ) ;
#5754=DIRECTION ( 'NONE',  ( 0.000000000000000000, 1.000000000000000000, 0.000000000000000000 ) ) ;
#5756=EDGE_CURVE ( 'NONE', #5029, #4261, #3336, .T. ) ;
#5757=ORIENTED_EDGE ( 'NONE', *, *, #2827, .T. ) ;
#5762=ORIENTED_EDGE ( 'NONE', *, *, #2090, .F. ) ;
#5763=CARTESIAN_POINT ( 'NONE',  ( 2.624999999999996891, -28.54166666666666785, 4.546633369868304797 ) ) ;
#5764=VECTOR ( 'NONE', #2723, 1000.000000000000000 ) ;
#5765=CARTESIAN_POINT ( 'NONE',  ( -2.557341765624999042, -27.33854166700806587, -4.429445870380400052 ) ) ;
#5767=CIRCLE ( 'NONE', #8164, 5.250000000000000000 ) ;
#5768=CARTESIAN_POINT ( 'NONE',  ( 5.114683531250000748, -27.67187500034139802, 0.000000000000000000 ) ) ;
#5769=CARTESIAN_POINT ( 'NONE',  ( 0.000000000000000000, 75.00000000000000000, 0.000000000000000000 ) ) ;
#5771=CARTESIAN_POINT ( 'NONE',  ( 9.180150650966086169E-15, -28.56249999999999645, 5.249999999999999112 ) ) ;
#5773=CARTESIAN_POINT ( 'NONE',  ( -2.557341765624999042, -29.58854166700806232, -4.429445870380400052 ) ) ;
#5779=CARTESIAN_POINT ( 'NONE',  ( -5.114683531249999859, -28.25520833367473017, -2.952963913586935440 ) ) ;
#5783=CARTESIAN_POINT ( 'NONE',  ( 6.972266317189433020E-16, -28.68749999999999645, -5.249999999999999112 ) ) ;
#5784=CARTESIAN_POINT ( 'NONE',  ( 2.033577675846918216E-14, -26.84375000068279959, 5.250000000000000888 ) ) ;
#5789=( BOUNDED_CURVE ( )  B_SPLINE_CURVE ( 2, ( #3682, #6505, #141, #2993, #8654, #6079, #4601, #1156, #1255 ),
 .UNSPECIFIED., .F., .F. ) 
 B_SPLINE_CURVE_WITH_KNOTS ( ( 3, 2, 2, 2, 3 ),
 ( 0.06250000000000000000, 0.06944444444444444753, 0.08333333333333332871, 0.09722222222222222376, 0.1041666666666666713 ),
 .UNSPECIFIED. ) 
 CURVE ( )  GEOMETRIC_REPRESENTATION_ITEM ( )  RATIONAL_B_SPLINE_CURVE ( ( 0.9330127018922194093, 0.9330127018922194093, 1.000000000000000000, 0.8660254037844387076, 1.000000000000000000, 0.8660254037844387076, 1.000000000000000000, 0.9330127018922192983, 0.9330127018922194093 ) ) 
 REPRESENTATION_ITEM ( '' )  );
#5791=CARTESIAN_POINT ( 'NONE',  ( -2.624999999999998668, -28.94791666734946389, -4.546633369868303021 ) ) ;
#5794=CARTESIAN_POINT ( 'NONE',  ( 5.114683531249999859, -27.58854166700806587, -2.952963913586932776 ) ) ;
#5797=DIRECTION ( 'NONE',  ( 0.000000000000000000, 1.000000000000000000, 0.000000000000000000 ) ) ;
#5800=ADVANCED_FACE ( 'NONE', ( #510 ), #4793, .T. ) ;
#5805=CARTESIAN_POINT ( 'NONE',  ( -5.250000000000000888, -27.85416666666666430, 3.031088913245533423 ) ) ;
#5814=ORIENTED_EDGE ( 'NONE', *, *, #5917, .F. ) ;
#5815=CARTESIAN_POINT ( 'NONE',  ( 5.249999999999999112, -28.77083333333333215, 3.031088913245538308 ) ) ;
#5817=CARTESIAN_POINT ( 'NONE',  ( -1.084901341431563726E-15, -28.48437500034139802, 5.905927827173866440 ) ) ;
#5819=CARTESIAN_POINT ( 'NONE',  ( -5.114683531250000748, -27.77604166700806587, 2.952963913586931888 ) ) ;
#5820=DIRECTION ( 'NONE',  ( -0.000000000000000000, -1.000000000000000000, -0.000000000000000000 ) ) ;
#5828=AXIS2_PLACEMENT_3D ( 'NONE', #2290, #3786, #6610 ) ;
#5829=CARTESIAN_POINT ( 'NONE',  ( -5.249999999999999112, -29.39583333333332860, -3.031088913245536975 ) ) ;
#5830=CARTESIAN_POINT ( 'NONE',  ( -5.114683531250000748, -28.48437500034139802, -6.263680815196995234E-16 ) ) ;
#5831=EDGE_CURVE ( 'NONE', #3312, #3105, #37, .T. ) ;
#5833=CARTESIAN_POINT ( 'NONE',  ( 2.033577675846918216E-14, -27.09375000068279604, 5.250000000000000888 ) ) ;
#5836=AXIS2_PLACEMENT_3D ( 'NONE', #2720, #7553, #5502 ) ;
#5838=ORIENTED_EDGE ( 'NONE', *, *, #3174, .F. ) ;
#5840=CARTESIAN_POINT ( 'NONE',  ( 2.624999999999996891, -29.57291666734946034, 4.546633369868304797 ) ) ;
#5842=AXIS2_PLACEMENT_3D ( 'NONE', #2972, #3070, #7380 ) ;
#5843=CARTESIAN_POINT ( 'NONE',  ( 2.557341765625000818, -29.88020833367473372, -4.429445870380400052 ) ) ;
#5844=DIRECTION ( 'NONE',  ( 0.000000000000000000, -0.000000000000000000, 1.000000000000000000 ) ) ;
#5848=AXIS2_PLACEMENT_3D ( 'NONE', #8765, #2396, #2208 ) ;
#5850=CARTESIAN_POINT ( 'NONE',  ( 6.972266317189433020E-16, -27.18750000000000000, -5.249999999999999112 ) ) ;
#5856=CARTESIAN_POINT ( 'NONE',  ( -1.406733260263385521, -27.32366454968462932, 5.250000000000006217 ) ) ;
#5861=CARTESIAN_POINT ( 'NONE',  ( 5.250000000000000000, -28.22916666666666430, -3.031088913245534755 ) ) ;
#5862=CARTESIAN_POINT ( 'NONE',  ( -2.557341765624999042, -28.08854166700806587, -4.429445870380400052 ) ) ;
#5863=FILL_AREA_STYLE_COLOUR ( '', #1299 ) ;
#5867=CARTESIAN_POINT ( 'NONE',  ( 0.000000000000000000, -30.00000000000000000, 0.000000000000000000 ) ) ;
#5870=( BOUNDED_CURVE ( )  B_SPLINE_CURVE ( 2, ( #5268, #7414, #8114, #2488, #6108, #8936, #8162, #3887, #2588 ),
 .UNSPECIFIED., .F., .T. ) 
 B_SPLINE_CURVE_WITH_KNOTS ( ( 3, 2, 2, 2, 3 ),
 ( 0.2291666666666666574, 0.2361111111111111049, 0.2500000000000000000, 0.2638888888888888951, 0.2708333333333333148 ),
 .UNSPECIFIED. ) 
 CURVE ( )  GEOMETRIC_REPRESENTATION_ITEM ( )  RATIONAL_B_SPLINE_CURVE ( ( 0.9330127018922194093, 0.9330127018922194093, 1.000000000000000000, 0.8660254037844387076, 1.000000000000000000, 0.8660254037844387076, 1.000000000000000000, 0.9330127018922196314, 0.9330127018922194093 ) ) 
 REPRESENTATION_ITEM ( '' )  );
#5871=CARTESIAN_POINT ( 'NONE',  ( 2.625000000000000444, -27.23958333401612819, -4.546633369868303021 ) ) ;
#5873=ORIENTED_EDGE ( 'NONE', *, *, #6326, .F. ) ;
#5875=CARTESIAN_POINT ( 'NONE',  ( -1.975475456537005874E-15, -29.31250000000000000, 5.250000000000000000 ) ) ;
#5876=CARTESIAN_POINT ( 'NONE',  ( -5.114683531250000748, -27.98437500034139802, -6.263680815196995234E-16 ) ) ;
#5882=CARTESIAN_POINT ( 'NONE',  ( 5.249999999999999112, -27.47916666666666430, -3.031088913245534755 ) ) ;
#5885=CARTESIAN_POINT ( 'NONE',  ( -5.250000000000000000, -28.90625000068279604, -6.429395695523604153E-16 ) ) ;
#5887=CARTESIAN_POINT ( 'NONE',  ( -1.084901341431563923E-15, -26.92187500034139802, 5.905927827173866440 ) ) ;
#5888=DIRECTION ( 'NONE',  ( 0.000000000000000000, 1.000000000000000000, 0.000000000000000000 ) ) ;
#5895=LINE ( 'NONE', #3812, #5682 ) ;
#5902=CARTESIAN_POINT ( 'NONE',  ( -5.249999999999999112, -27.39583333333333215, -3.031088913245536975 ) ) ;
#5903=EDGE_LOOP ( 'NONE', ( #9174, #4737 ) ) ;
#5907=CARTESIAN_POINT ( 'NONE',  ( 2.625000000000000444, -27.20833333333333215, -4.546633369868303021 ) ) ;
#5909=CARTESIAN_POINT ( 'NONE',  ( 2.557341765625000818, -27.63020833367473017, -4.429445870380400052 ) ) ;
#5911=CARTESIAN_POINT ( 'NONE',  ( 5.114683531249998971, -26.94270833367472662, 2.952963913586936329 ) ) ;
#5916=CARTESIAN_POINT ( 'NONE',  ( -2.557341765625002594, -28.25520833367473017, 4.429445870380399164 ) ) ;
#5917=EDGE_CURVE ( 'NONE', #3802, #7275, #8236, .T. ) ;
#5918=ORIENTED_EDGE ( 'NONE', *, *, #6113, .T. ) ;
#5920=CARTESIAN_POINT ( 'NONE',  ( 3.616337804771879580E-16, -28.29687500034139802, -5.905927827173866440 ) ) ;
#5921=AXIS2_PLACEMENT_3D ( 'NONE', #7535, #1873, #1298 ) ;
#5925=FACE_OUTER_BOUND ( 'NONE', #1656, .T. ) ;
#5926=CARTESIAN_POINT ( 'NONE',  ( 0.000000000000000000, -30.00000000000000000, 5.250000000000000000 ) ) ;
#5928=CARTESIAN_POINT ( 'NONE',  ( -5.250000000000000000, -29.12499999999999645, -6.429395695523604153E-16 ) ) ;
#5930=ORIENTED_EDGE ( 'NONE', *, *, #5548, .T. ) ;
#5932=CARTESIAN_POINT ( 'NONE',  ( -5.250000000000000888, -29.13541666734946389, 3.031088913245532979 ) ) ;
#5935=CARTESIAN_POINT ( 'NONE',  ( 3.616337804771879580E-16, -27.79687500034139802, -5.905927827173866440 ) ) ;
#5936=ORIENTED_EDGE ( 'NONE', *, *, #79, .T. ) ;
#5937=CARTESIAN_POINT ( 'NONE',  ( 0.000000000000000000, -30.00000000000000000, 0.000000000000000000 ) ) ;
#5943=VECTOR ( 'NONE', #3594, 1000.000000000000000 ) ;
#5946=CARTESIAN_POINT ( 'NONE',  ( 0.000000000000000000, -30.00000000000000000, 0.000000000000000000 ) ) ;
#5951=VERTEX_POINT ( 'NONE', #5572 ) ;
#5955=CARTESIAN_POINT ( 'NONE',  ( -2.625000000000002220, -27.58333333333333215, 4.546633369868302132 ) ) ;
#5961=CARTESIAN_POINT ( 'NONE',  ( -5.114683531250000748, -28.48437500034139802, -6.263680815196995234E-16 ) ) ;
#5963=CARTESIAN_POINT ( 'NONE',  ( 5.249999999999999112, -28.51041666734946389, -3.031088913245534755 ) ) ;
#5964=CARTESIAN_POINT ( 'NONE',  ( -1.406733260263382856, -27.45758545099817027, -5.250000000000006217 ) ) ;
#5965=CARTESIAN_POINT ( 'NONE',  ( -5.114683531249999859, -29.31770833367473372, -2.952963913586935440 ) ) ;
#5968=ORIENTED_EDGE ( 'NONE', *, *, #3959, .F. ) ;
#5999=CARTESIAN_POINT ( 'NONE',  ( -5.250000000000000000, -28.39583333333333215, -3.031088913245536531 ) ) ;
#6005=CARTESIAN_POINT ( 'NONE',  ( 3.616337804771879580E-16, -29.54687500034139802, -5.905927827173866440 ) ) ;
#6009=CARTESIAN_POINT ( 'NONE',  ( 2.557341765624996821, -28.21354166700806587, 4.429445870380401828 ) ) ;
#6012=CARTESIAN_POINT ( 'NONE',  ( -5.114683531250000748, -27.73437500034139802, -6.263680815196995234E-16 ) ) ;
#6013=EDGE_CURVE ( 'NONE', #1550, #3111, #2239, .T. ) ;
#6015=CARTESIAN_POINT ( 'NONE',  ( 7.041719095097280880E-16, -9.000000000000000000, -5.750000000000000000 ) ) ;
#6018=CARTESIAN_POINT ( 'NONE',  ( 5.249999999999999112, -29.97916666666666430, -3.031088913245534755 ) ) ;
#6022=CARTESIAN_POINT ( 'NONE',  ( -1.113604000661152470E-15, -27.59375000068279959, 6.062177826491070398 ) ) ;
#6028=CARTESIAN_POINT ( 'NONE',  ( 6.429395695523604153E-16, -30.00000000000000000, -5.250000000000000000 ) ) ;
#6031=CARTESIAN_POINT ( 'NONE',  ( -1.084901341431563923E-15, -29.42187500034139447, 5.905927827173866440 ) ) ;
#6036=FACE_OUTER_BOUND ( 'NONE', #519, .T. ) ;
#6041=CARTESIAN_POINT ( 'NONE',  ( -2.624999999999998668, -27.66666666666666430, -4.546633369868303021 ) ) ;
#6046=ORIENTED_EDGE ( 'NONE', *, *, #1730, .T. ) ;
#6049=CARTESIAN_POINT ( 'NONE',  ( 5.114683531250000748, -29.10937500034139802, 0.000000000000000000 ) ) ;
#6053=CARTESIAN_POINT ( 'NONE',  ( -1.084901341431563923E-15, -28.98437500034139447, 5.905927827173866440 ) ) ;
#6057=CARTESIAN_POINT ( 'NONE',  ( -1.406733260263382856, -27.95758545099817027, -5.250000000000006217 ) ) ;
#6058=LINE ( 'NONE', #7604, #1049 ) ;
#6059=EDGE_CURVE ( 'NONE', #5951, #1550, #5504, .T. ) ;
#6060=ORIENTED_EDGE ( 'NONE', *, *, #222, .T. ) ;
#6064=DIRECTION ( 'NONE',  ( 0.000000000000000000, 1.000000000000000000, 0.000000000000000000 ) ) ;
#6069=CARTESIAN_POINT ( 'NONE',  ( 3.712013335537174572E-16, -28.21875000068279604, -6.062177826491070398 ) ) ;
#6075=FACE_BOUND ( 'NONE', #5903, .T. ) ;
#6077=CIRCLE ( 'NONE', #8015, 5.750000000000000000 ) ;
#6079=CARTESIAN_POINT ( 'NONE',  ( 5.249999999999999112, -29.72916666666666430, -3.031088913245534755 ) ) ;
#6081=AXIS2_PLACEMENT_3D ( 'NONE', #8175, #3384, #2689 ) ;
#6086=DIRECTION ( 'NONE',  ( -0.000000000000000000, -1.000000000000000000, -0.000000000000000000 ) ) ;
#6091=ORIENTED_EDGE ( 'NONE', *, *, #5756, .T. ) ;
#6092=DIRECTION ( 'NONE',  ( 0.000000000000000000, 0.000000000000000000, 1.000000000000000000 ) ) ;
#6094=FACE_OUTER_BOUND ( 'NONE', #1883, .T. ) ;
#6102=CARTESIAN_POINT ( 'NONE',  ( 2.557341765625000818, -29.56770833367473017, -4.429445870380400052 ) ) ;
#6105=CARTESIAN_POINT ( 'NONE',  ( 5.114683531249998971, -28.69270833367473017, 2.952963913586936329 ) ) ;
#6107=ADVANCED_FACE ( 'NONE', ( #1710 ), #8083, .T. ) ;
#6108=CARTESIAN_POINT ( 'NONE',  ( 5.250000000000000000, -29.25000000000000000, 0.000000000000000000 ) ) ;
#6109=CIRCLE ( 'NONE', #5360, 4.250000000000000000 ) ;
#6110=DIRECTION ( 'NONE',  ( 0.000000000000000000, 1.000000000000000000, 0.000000000000000000 ) ) ;
#6112=CARTESIAN_POINT ( 'NONE',  ( -5.114683531250000748, -28.52604166700806587, 2.952963913586931888 ) ) ;
#6113=EDGE_CURVE ( 'NONE', #4963, #4350, #5396, .T. ) ;
#6116=CARTESIAN_POINT ( 'NONE',  ( -1.406733260263393293, -29.20758545099816317, -5.250000000000000000 ) ) ;
#6122=CARTESIAN_POINT ( 'NONE',  ( -2.624999999999998668, -27.69791666734946389, -4.546633369868303021 ) ) ;
#6124=ORIENTED_EDGE ( 'NONE', *, *, #8283, .F. ) ;
#6128=ADVANCED_FACE ( 'NONE', ( #218 ), #124, .T. ) ;
#6129=CARTESIAN_POINT ( 'NONE',  ( -1.406733260263390628, -28.82366454968462577, 5.250000000000001776 ) ) ;
#6130=CYLINDRICAL_SURFACE ( 'NONE', #3766, 5.250000000000000000 ) ;
#6133=CARTESIAN_POINT ( 'NONE',  ( 3.616337804771879580E-16, -29.29687500034139447, -5.905927827173866440 ) ) ;
#6134=FACE_OUTER_BOUND ( 'NONE', #1457, .T. ) ;
#6137=EDGE_CURVE ( 'NONE', #8090, #1056, #794, .T. ) ;
#6144=ORIENTED_EDGE ( 'NONE', *, *, #8067, .F. ) ;
#6145=CARTESIAN_POINT ( 'NONE',  ( -2.625000000000002220, -27.11458333401612819, 4.546633369868302132 ) ) ;
#6146=DIRECTION ( 'NONE',  ( 0.000000000000000000, 0.000000000000000000, 1.000000000000000000 ) ) ;
#6147=CARTESIAN_POINT ( 'NONE',  ( 5.114683531249998971, -27.19270833367473017, 2.952963913586936329 ) ) ;
#6149=ORIENTED_EDGE ( 'NONE', *, *, #2638, .F. ) ;
#6153=CARTESIAN_POINT ( 'NONE',  ( 2.557341765624996821, -28.65104166700806587, 4.429445870380401828 ) ) ;
#6155=DIRECTION ( 'NONE',  ( 0.000000000000000000, 0.000000000000000000, 1.000000000000000000 ) ) ;
#6156=CARTESIAN_POINT ( 'NONE',  ( 2.557341765624996821, -27.71354166700806587, 4.429445870380401828 ) ) ;
#6160=CARTESIAN_POINT ( 'NONE',  ( 5.114683531250000748, -29.92187500034139802, 0.000000000000000000 ) ) ;
#6162=CARTESIAN_POINT ( 'NONE',  ( 5.114683531249999859, -29.65104166700806232, -2.952963913586932776 ) ) ;
#6165=PLANE ( 'NONE',  #6569 ) ;
#6170=ORIENTED_EDGE ( 'NONE', *, *, #1794, .T. ) ;
#6171=CYLINDRICAL_SURFACE ( 'NONE', #6081, 5.250000000000000000 ) ;
#6172=CARTESIAN_POINT ( 'NONE',  ( 5.249999999999999112, -28.30208333401612819, 3.031088913245538308 ) ) ;
#6178=CARTESIAN_POINT ( 'NONE',  ( 5.249999999999997335, -29.52083333333333215, 3.031088913245538308 ) ) ;
#6192=CARTESIAN_POINT ( 'NONE',  ( -1.113604000661152470E-15, -27.06250000000000000, 6.062177826491070398 ) ) ;
#6198=CARTESIAN_POINT ( 'NONE',  ( 3.616337804771879580E-16, -27.29687500034139802, -5.905927827173866440 ) ) ;
#6201=CARTESIAN_POINT ( 'NONE',  ( 5.114683531249999859, -27.40104166700806587, -2.952963913586932776 ) ) ;
#6202=CARTESIAN_POINT ( 'NONE',  ( 1.406733260263405061, -27.22991455036742536, -5.249999999999994671 ) ) ;
#6203=CARTESIAN_POINT ( 'NONE',  ( 5.114683531250000748, -29.17187500034139802, 0.000000000000000000 ) ) ;
#6204=CARTESIAN_POINT ( 'NONE',  ( -5.249999999999999112, -28.39583333333333215, -3.031088913245536975 ) ) ;
#6205=CARTESIAN_POINT ( 'NONE',  ( -1.084901341431563923E-15, -29.48437500034139802, 5.905927827173866440 ) ) ;
#6215=ORIENTED_EDGE ( 'NONE', *, *, #8454, .F. ) ;
#6217=CARTESIAN_POINT ( 'NONE',  ( 5.250000000000000000, -27.76041666734946389, -3.031088913245534755 ) ) ;
#6227=CARTESIAN_POINT ( 'NONE',  ( 2.557341765625000818, -29.06770833367473017, -4.429445870380400052 ) ) ;
#6228=CARTESIAN_POINT ( 'NONE',  ( 5.249999999999997335, -27.55208333401612819, 3.031088913245538308 ) ) ;
#6232=CARTESIAN_POINT ( 'NONE',  ( 5.250000000000000000, -27.00000000000000000, 0.000000000000000000 ) ) ;
#6236=CARTESIAN_POINT ( 'NONE',  ( -2.624999999999998668, -27.16666666666666430, -4.546633369868303021 ) ) ;
#6237=LINE ( 'NONE', #4058, #8336 ) ;
#6239=EDGE_LOOP ( 'NONE', ( #158, #235, #7390, #7476 ) ) ;
#6241=CARTESIAN_POINT ( 'NONE',  ( 5.114683531250000748, -27.60937500034139802, 0.000000000000000000 ) ) ;
#6244=AXIS2_PLACEMENT_3D ( 'NONE', #8057, #5820, #4476 ) ;
#6245=CARTESIAN_POINT ( 'NONE',  ( -5.250000000000000000, -29.87500000000000000, -6.429395695523604153E-16 ) ) ;
#6247=AXIS2_PLACEMENT_3D ( 'NONE', #8278, #4692, #3863 ) ;
#6248=CARTESIAN_POINT ( 'NONE',  ( 5.114683531250000748, -28.65104166700806587, -2.952963913586932776 ) ) ;
#6250=CARTESIAN_POINT ( 'NONE',  ( -2.557341765625002594, -29.25520833367473017, 4.429445870380399164 ) ) ;
#6254=CARTESIAN_POINT ( 'NONE',  ( 2.625000000000000444, -29.48958333401613174, -4.546633369868303021 ) ) ;
#6258=VERTEX_POINT ( 'NONE', #2694 ) ;
#6261=CARTESIAN_POINT ( 'NONE',  ( -5.114683531250000748, -29.46354166700806232, 2.952963913586931888 ) ) ;
#6269=CARTESIAN_POINT ( 'NONE',  ( 5.114683531250000748, -28.60937500034139802, 0.000000000000000000 ) ) ;
#6277=DIRECTION ( 'NONE',  ( 0.000000000000000000, 1.000000000000000000, 0.000000000000000000 ) ) ;
#6278=CARTESIAN_POINT ( 'NONE',  ( 9.180150650966086169E-15, -28.59375000068279959, 5.250000000000000000 ) ) ;
#6283=CARTESIAN_POINT ( 'NONE',  ( 5.114683531249998971, -27.88020833367473017, 2.952963913586936329 ) ) ;
#6285=CARTESIAN_POINT ( 'NONE',  ( 2.557341765624996821, -26.96354166700806232, 4.429445870380401828 ) ) ;
#6289=CARTESIAN_POINT ( 'NONE',  ( -2.557341765624999042, -28.83854166700806587, -4.429445870380400052 ) ) ;
#6290=CARTESIAN_POINT ( 'NONE',  ( -2.557341765625002594, -28.50520833367473017, 4.429445870380399164 ) ) ;
#6295=CARTESIAN_POINT ( 'NONE',  ( 5.249999999999999112, -28.47916666666666785, -3.031088913245534755 ) ) ;
#6300=CARTESIAN_POINT ( 'NONE',  ( 2.625000000000000444, -26.98958333401612819, -4.546633369868303021 ) ) ;
#6305=CARTESIAN_POINT ( 'NONE',  ( -1.406733260263385521, -27.07366454968463287, 5.250000000000006217 ) ) ;
#6310=CARTESIAN_POINT ( 'NONE',  ( -2.557341765624999042, -29.02604166700806587, -4.429445870380400052 ) ) ;
#6318=ORIENTED_EDGE ( 'NONE', *, *, #1165, .T. ) ;
#6322=CARTESIAN_POINT ( 'NONE',  ( -2.557341765625002594, -27.94270833367473017, 4.429445870380399164 ) ) ;
#6324=CARTESIAN_POINT ( 'NONE',  ( 5.114683531249999859, -27.65104166700806232, -2.952963913586932776 ) ) ;
#6326=EDGE_CURVE ( 'NONE', #566, #8116, #7369, .T. ) ;
#6327=CARTESIAN_POINT ( 'NONE',  ( 2.557341765624996821, -28.71354166700806587, 4.429445870380401828 ) ) ;
#6329=CARTESIAN_POINT ( 'NONE',  ( -1.084901341431563923E-15, -27.98437500034139802, 5.905927827173866440 ) ) ;
#6340=CARTESIAN_POINT ( 'NONE',  ( 2.557341765624996821, -29.40104166700806232, 4.429445870380401828 ) ) ;
#6341=EDGE_CURVE ( 'NONE', #4820, #1374, #3846, .T. ) ;
#6342=( GEOMETRIC_REPRESENTATION_CONTEXT ( 3 ) GLOBAL_UNCERTAINTY_ASSIGNED_CONTEXT ( ( #3763 ) ) GLOBAL_UNIT_ASSIGNED_CONTEXT ( ( #145, #7872, #3546 ) ) REPRESENTATION_CONTEXT ( 'NONE', 'WORKASPACE' ) );
#6346=CARTESIAN_POINT ( 'NONE',  ( -1.975475456537005874E-15, -28.09375000068279604, 5.249999999999999112 ) ) ;
#6347=ORIENTED_EDGE ( 'NONE', *, *, #2711, .T. ) ;
#6349=CARTESIAN_POINT ( 'NONE',  ( 0.000000000000000000, -9.999999999999998224, 2.750000000000000000 ) ) ;
#6352=CARTESIAN_POINT ( 'NONE',  ( -2.557341765625002594, -28.94270833367473017, 4.429445870380399164 ) ) ;
#6356=CARTESIAN_POINT ( 'NONE',  ( -1.975475456537005874E-15, -28.09375000068279604, 5.250000000000000000 ) ) ;
#6361=CARTESIAN_POINT ( 'NONE',  ( -1.406733260263393293, -26.95758545099816672, -5.250000000000000000 ) ) ;
#6365=CARTESIAN_POINT ( 'NONE',  ( -5.114683531250000748, -27.48437500034139802, -6.263680815196995234E-16 ) ) ;
#6367=CARTESIAN_POINT ( 'NONE',  ( 5.249999999999999112, -29.52083333333333215, 3.031088913245538308 ) ) ;
#6369=CARTESIAN_POINT ( 'NONE',  ( 2.557341765625000818, -29.38020833367473017, -4.429445870380400052 ) ) ;
#6370=CARTESIAN_POINT ( 'NONE',  ( -5.114683531250000748, -27.04687500034139802, -6.263680815196995234E-16 ) ) ;
#6372=CARTESIAN_POINT ( 'NONE',  ( -5.249999999999999112, -28.42708333401612819, -3.031088913245536975 ) ) ;
#6377=CARTESIAN_POINT ( 'NONE',  ( -2.557341765624999042, -29.83854166700806232, -4.429445870380400052 ) ) ;
#6380=ORIENTED_EDGE ( 'NONE', *, *, #3497, .T. ) ;
#6383=CARTESIAN_POINT ( 'NONE',  ( 5.114683531250000748, -29.60937500034139802, 0.000000000000000000 ) ) ;
#6384=( BOUNDED_CURVE ( )  B_SPLINE_CURVE ( 2, ( #4117, #3425, #4529, #984, #5217, #7217, #7265, #6564, #3000 ),
 .UNSPECIFIED., .F., .F. ) 
 B_SPLINE_CURVE_WITH_KNOTS ( ( 3, 2, 2, 2, 3 ),
 ( 0.3125000000000000000, 0.3194444444444444198, 0.3333333333333333148, 0.3472222222222222099, 0.3541666666666666297 ),
 .UNSPECIFIED. ) 
 CURVE ( )  GEOMETRIC_REPRESENTATION_ITEM ( )  RATIONAL_B_SPLINE_CURVE ( ( 0.9330127018922194093, 0.9330127018922194093, 1.000000000000000000, 0.8660254037844387076, 1.000000000000000000, 0.8660254037844387076, 1.000000000000000000, 0.9330127018922196314, 0.9330127018922194093 ) ) 
 REPRESENTATION_ITEM ( '' )  );
#6385=ADVANCED_FACE ( 'NONE', ( #3009 ), #1699, .T. ) ;
#6391=VECTOR ( 'NONE', #1606, 1000.000000000000000 ) ;
#6392=EDGE_CURVE ( 'NONE', #4680, #784, #2256, .T. ) ;
#6397=CARTESIAN_POINT ( 'NONE',  ( -5.114683531250000748, -28.48437500034139802, -6.263680815196995234E-16 ) ) ;
#6402=FACE_OUTER_BOUND ( 'NONE', #2114, .T. ) ;
#6406=ADVANCED_FACE ( 'NONE', ( #5925 ), #993, .T. ) ;
#6409=EDGE_LOOP ( 'NONE', ( #3729, #6835 ) ) ;
#6413=CARTESIAN_POINT ( 'NONE',  ( -2.625000000000002220, -29.33333333333333215, 4.546633369868302132 ) ) ;
#6415=CARTESIAN_POINT ( 'NONE',  ( -5.114683531250000748, -27.81770833367473017, -2.952963913586935440 ) ) ;
#6416=VECTOR ( 'NONE', #4784, 1000.000000000000000 ) ;
#6418=CARTESIAN_POINT ( 'NONE',  ( 5.114683531249999859, -27.90104166700806587, -2.952963913586932776 ) ) ;
#6423=CARTESIAN_POINT ( 'NONE',  ( 2.625000000000000444, -28.45833333333333215, -4.546633369868303021 ) ) ;
#6429=CARTESIAN_POINT ( 'NONE',  ( 5.249999999999999112, -27.05208333401612819, 3.031088913245538308 ) ) ;
#6430=VERTEX_POINT ( 'NONE', #5833 ) ;
#6432=EDGE_LOOP ( 'NONE', ( #3647, #6982, #8902 ) ) ;
#6435=CARTESIAN_POINT ( 'NONE',  ( 6.972266317189433020E-16, -27.18750000000000000, -5.250000000000000000 ) ) ;
#6441=CARTESIAN_POINT ( 'NONE',  ( 5.249999999999999112, -27.76041666734946389, -3.031088913245534755 ) ) ;
#6442=CARTESIAN_POINT ( 'NONE',  ( -1.084901341431563923E-15, -27.92187500034139802, 5.905927827173866440 ) ) ;
#6451=CYLINDRICAL_SURFACE ( 'NONE', #4898, 5.250000000000000000 ) ;
#6452=EDGE_LOOP ( 'NONE', ( #6795, #6648, #460, #3941 ) ) ;
#6454=VERTEX_POINT ( 'NONE', #5783 ) ;
#6457=EDGE_CURVE ( 'NONE', #7180, #2870, #7041, .T. ) ;
#6459=CARTESIAN_POINT ( 'NONE',  ( -5.250000000000000888, -28.60416666666666430, 3.031088913245532979 ) ) ;
#6462=CARTESIAN_POINT ( 'NONE',  ( 2.557341765625000818, -27.38020833367473017, -4.429445870380400052 ) ) ;
#6463=CARTESIAN_POINT ( 'NONE',  ( -2.557341765625002594, -28.25520833367473017, 4.429445870380399164 ) ) ;
#6465=DIRECTION ( 'NONE',  ( 1.000000000000000000, 0.000000000000000000, 0.000000000000000000 ) ) ;
#6468=CARTESIAN_POINT ( 'NONE',  ( -5.114683531250000748, -29.79687500034139802, -6.263680815196995234E-16 ) ) ;
#6472=CARTESIAN_POINT ( 'NONE',  ( 2.625000000000000444, -27.95833333333333215, -4.546633369868303021 ) ) ;
#6473=CARTESIAN_POINT ( 'NONE',  ( 3.616337804771879580E-16, -27.79687500034139802, -5.905927827173866440 ) ) ;
#6482=CARTESIAN_POINT ( 'NONE',  ( 6.972266317189433020E-16, -29.93750000000000000, -5.250000000000000000 ) ) ;
#6483=CARTESIAN_POINT ( 'NONE',  ( 5.249999999999999112, -29.05208333401612819, 3.031088913245538308 ) ) ;
#6486=CARTESIAN_POINT ( 'NONE',  ( -2.557341765625002594, -26.94270833367473017, 4.429445870380399164 ) ) ;
#6488=DIRECTION ( 'NONE',  ( -0.000000000000000000, -1.000000000000000000, -0.000000000000000000 ) ) ;
#6490=CARTESIAN_POINT ( 'NONE',  ( -5.249999999999999112, -28.17708333401612819, -3.031088913245536975 ) ) ;
#6494=DIRECTION ( 'NONE',  ( 0.000000000000000000, -0.000000000000000000, 1.000000000000000000 ) ) ;
#6495=DIRECTION ( 'NONE',  ( 0.000000000000000000, 1.000000000000000000, 0.000000000000000000 ) ) ;
#6499=VERTEX_POINT ( 'NONE', #4582 ) ;
#6503=CARTESIAN_POINT ( 'NONE',  ( -5.250000000000000000, -29.12499999999999645, -6.429395695523604153E-16 ) ) ;
#6505=CARTESIAN_POINT ( 'NONE',  ( 1.406733260263391960, -29.80133545031536713, 5.250000000000000000 ) ) ;
#6507=CARTESIAN_POINT ( 'NONE',  ( 2.557341765625000818, -28.13020833367473017, -4.429445870380400052 ) ) ;
#6510=CARTESIAN_POINT ( 'NONE',  ( 2.557341765625000818, -27.38020833367473017, -4.429445870380400052 ) ) ;
#6511=DIRECTION ( 'NONE',  ( 0.000000000000000000, 0.000000000000000000, 1.000000000000000000 ) ) ;
#6517=CARTESIAN_POINT ( 'NONE',  ( 5.249999999999997335, -28.30208333401612819, 3.031088913245538308 ) ) ;
#6518=ORIENTED_EDGE ( 'NONE', *, *, #8818, .T. ) ;
#6521=CARTESIAN_POINT ( 'NONE',  ( 5.249999999999997335, -28.02083333333333215, 3.031088913245538308 ) ) ;
#6522=CARTESIAN_POINT ( 'NONE',  ( 5.114683531250000748, -29.10937500034139802, 0.000000000000000000 ) ) ;
#6525=AXIS2_PLACEMENT_3D ( 'NONE', #484, #8987, #2635 ) ;
#6529=VERTEX_POINT ( 'NONE', #6015 ) ;
#6532=CARTESIAN_POINT ( 'NONE',  ( -5.250000000000000000, -29.65625000068279604, -6.429395695523604153E-16 ) ) ;
#6535=CARTESIAN_POINT ( 'NONE',  ( 5.114683531250000748, -29.92187500034139802, 0.000000000000000000 ) ) ;
#6540=DIRECTION ( 'NONE',  ( 0.000000000000000000, 1.000000000000000000, 0.000000000000000000 ) ) ;
#6541=CIRCLE ( 'NONE', #4207, 5.250000000000000000 ) ;
#6556=ORIENTED_EDGE ( 'NONE', *, *, #1538, .T. ) ;
#6557=CARTESIAN_POINT ( 'NONE',  ( 5.250000000000000000, -27.75000000000000000, 0.000000000000000000 ) ) ;
#6559=CARTESIAN_POINT ( 'NONE',  ( 2.557341765624996821, -27.21354166700806587, 4.429445870380401828 ) ) ;
#6561=CARTESIAN_POINT ( 'NONE',  ( -1.975475456537005874E-15, -29.34375000068279249, 5.250000000000000000 ) ) ;
#6562=CARTESIAN_POINT ( 'NONE',  ( -5.114683531250000748, -29.75520833367473017, -2.952963913586935440 ) ) ;
#6564=CARTESIAN_POINT ( 'NONE',  ( 1.406733260263400176, -28.72991455036743602, -5.249999999999997335 ) ) ;
#6566=CARTESIAN_POINT ( 'NONE',  ( -1.084901341431563923E-15, -29.73437500034140157, 5.905927827173866440 ) ) ;
#6567=ORIENTED_EDGE ( 'NONE', *, *, #6457, .F. ) ;
#6569=AXIS2_PLACEMENT_3D ( 'NONE', #8991, #8306, #1938 ) ;
#6570=CARTESIAN_POINT ( 'NONE',  ( -2.625000000000002220, -29.33333333333333215, 4.546633369868302132 ) ) ;
#6571=CARTESIAN_POINT ( 'NONE',  ( -5.114683531250000748, -28.21354166700806232, 2.952963913586931888 ) ) ;
#6580=CARTESIAN_POINT ( 'NONE',  ( 2.300847884672513123E-14, -27.43750000000000355, -5.250000000000000000 ) ) ;
#6582=ORIENTED_EDGE ( 'NONE', *, *, #8142, .F. ) ;
#6584=AXIS2_PLACEMENT_3D ( 'NONE', #2412, #5100, #7387 ) ;
#6585=CARTESIAN_POINT ( 'NONE',  ( -5.250000000000000000, -29.15625000068279604, -6.429395695523604153E-16 ) ) ;
#6588=CARTESIAN_POINT ( 'NONE',  ( -5.114683531249999859, -27.75520833367473017, -2.952963913586935440 ) ) ;
#6594=AXIS2_PLACEMENT_3D ( 'NONE', #2305, #4440, #4718 ) ;
#6602=FACE_OUTER_BOUND ( 'NONE', #5257, .T. ) ;
#6603=ORIENTED_EDGE ( 'NONE', *, *, #6793, .T. ) ;
#6607=CARTESIAN_POINT ( 'NONE',  ( 5.250000000000000000, -27.25000000000000000, 0.000000000000000000 ) ) ;
#6608=CARTESIAN_POINT ( 'NONE',  ( 2.557341765625000818, -28.38020833367473017, -4.429445870380400052 ) ) ;
#6610=DIRECTION ( 'NONE',  ( 0.000000000000000000, 0.000000000000000000, 1.000000000000000000 ) ) ;
#6614=CARTESIAN_POINT ( 'NONE',  ( 2.625000000000000444, -28.70833333333333215, -4.546633369868303021 ) ) ;
#6615=CARTESIAN_POINT ( 'NONE',  ( -5.114683531250000748, -28.29687500034139447, -6.263680815196995234E-16 ) ) ;
#6616=CARTESIAN_POINT ( 'NONE',  ( 9.180150650966086169E-15, -28.34375000068279604, 5.250000000000000000 ) ) ;
#6618=CARTESIAN_POINT ( 'NONE',  ( 9.180150650966086169E-15, -28.34375000068279604, 5.249999999999999112 ) ) ;
#6619=CARTESIAN_POINT ( 'NONE',  ( -1.084901341431563923E-15, -28.42187500034139802, 5.905927827173866440 ) ) ;
#6620=ORIENTED_EDGE ( 'NONE', *, *, #4928, .T. ) ;
#6625=CARTESIAN_POINT ( 'NONE',  ( -1.975475456537005874E-15, -29.06249999999999645, 5.250000000000000000 ) ) ;
#6626=ORIENTED_EDGE ( 'NONE', *, *, #6672, .T. ) ;
#6628=DIRECTION ( 'NONE',  ( 0.000000000000000000, 0.000000000000000000, 1.000000000000000000 ) ) ;
#6629=CARTESIAN_POINT ( 'NONE',  ( 3.712013335537174572E-16, -28.71875000068279604, -6.062177826491070398 ) ) ;
#6631=CARTESIAN_POINT ( 'NONE',  ( -2.557341765625002594, -27.94270833367473017, 4.429445870380399164 ) ) ;
#6640=CARTESIAN_POINT ( 'NONE',  ( 2.625000000000000444, -27.70833333333333215, -4.546633369868303021 ) ) ;
#6648=ORIENTED_EDGE ( 'NONE', *, *, #698, .T. ) ;
#6649=CARTESIAN_POINT ( 'NONE',  ( -1.113604000661152470E-15, -27.56250000000000000, 6.062177826491070398 ) ) ;
#6654=CARTESIAN_POINT ( 'NONE',  ( 2.557341765624996821, -29.15104166700806587, 4.429445870380401828 ) ) ;
#6656=FACE_OUTER_BOUND ( 'NONE', #5224, .T. ) ;
#6657=CARTESIAN_POINT ( 'NONE',  ( 9.180150650966086169E-15, -28.81250000000000000, 5.250000000000000000 ) ) ;
#6658=CARTESIAN_POINT ( 'NONE',  ( 3.616337804771879580E-16, -28.60937500034139802, -5.905927827173866440 ) ) ;
#6659=CARTESIAN_POINT ( 'NONE',  ( 2.033577675846918216E-14, -27.06250000000000355, 5.250000000000000888 ) ) ;
#6662=CARTESIAN_POINT ( 'NONE',  ( 5.114683531249998971, -28.13020833367473017, 2.952963913586936329 ) ) ;
#6671=ORIENTED_EDGE ( 'NONE', *, *, #4478, .T. ) ;
#6672=EDGE_CURVE ( 'NONE', #2870, #5029, #2637, .T. ) ;
#6674=CARTESIAN_POINT ( 'NONE',  ( 2.625000000000000444, -29.73958333401613174, -4.546633369868303021 ) ) ;
#6679=EDGE_CURVE ( 'NONE', #874, #7322, #9181, .T. ) ;
#6690=ORIENTED_EDGE ( 'NONE', *, *, #672, .F. ) ;
#6695=CARTESIAN_POINT ( 'NONE',  ( -2.624999999999998668, -28.41666666666666785, -4.546633369868303021 ) ) ;
#6697=CARTESIAN_POINT ( 'NONE',  ( -2.557341765624999042, -27.08854166700806232, -4.429445870380400052 ) ) ;
#6700=CARTESIAN_POINT ( 'NONE',  ( -1.406733260263395735, -29.35491455036742892, 5.250000000000000000 ) ) ;
#6702=CARTESIAN_POINT ( 'NONE',  ( 5.114683531249998971, -28.88020833367473017, 2.952963913586936329 ) ) ;
#6704=CARTESIAN_POINT ( 'NONE',  ( 3.367778697655221012E-16, -9.999999999999998224, -2.750000000000000000 ) ) ;
#6705=DIRECTION ( 'NONE',  ( 0.000000000000000000, 1.000000000000000000, 0.000000000000000000 ) ) ;
#6706=CARTESIAN_POINT ( 'NONE',  ( -1.084901341431563923E-15, -28.48437500034139802, 5.905927827173866440 ) ) ;
#6708=CARTESIAN_POINT ( 'NONE',  ( 2.300847884672513123E-14, -27.46875000068279604, -5.250000000000000000 ) ) ;
#6709=CARTESIAN_POINT ( 'NONE',  ( 0.000000000000000000, -30.00000000000000000, 5.250000000000000000 ) ) ;
#6717=CARTESIAN_POINT ( 'NONE',  ( 5.249999999999999112, -28.55208333401613174, 3.031088913245538308 ) ) ;
#6720=VECTOR ( 'NONE', #1929, 1000.000000000000000 ) ;
#6724=CARTESIAN_POINT ( 'NONE',  ( 0.000000000000000000, 75.00000000000000000, 0.000000000000000000 ) ) ;
#6725=EDGE_CURVE ( 'NONE', #8837, #3172, #8940, .T. ) ;
#6726=VECTOR ( 'NONE', #3619, 1000.000000000000000 ) ;
#6729=CARTESIAN_POINT ( 'NONE',  ( 1.185285273922203525E-14, -28.71875000068279959, -5.249999999999999112 ) ) ;
#6731=CARTESIAN_POINT ( 'NONE',  ( -5.114683531249999859, -29.50520833367473017, -2.952963913586935440 ) ) ;
#6742=VERTEX_POINT ( 'NONE', #4890 ) ;
#6743=CARTESIAN_POINT ( 'NONE',  ( -2.624999999999998668, -28.16666666666666785, -4.546633369868303021 ) ) ;
#6749=SURFACE_STYLE_USAGE ( .BOTH. , #2432 ) ;
#6753=CARTESIAN_POINT ( 'NONE',  ( 5.114683531250000748, -28.35937500034139447, 0.000000000000000000 ) ) ;
#6755=CARTESIAN_POINT ( 'NONE',  ( 1.185285273922203525E-14, -28.93749999999999645, -5.249999999999999112 ) ) ;
#6757=CARTESIAN_POINT ( 'NONE',  ( 2.557341765625000818, -28.88020833367473017, -4.429445870380400052 ) ) ;
#6758=CARTESIAN_POINT ( 'NONE',  ( 0.000000000000000000, -30.00000000000000000, 0.000000000000000000 ) ) ;
#6760=CARTESIAN_POINT ( 'NONE',  ( -5.114683531250000748, -27.21354166700806587, 2.952963913586931888 ) ) ;
#6764=CARTESIAN_POINT ( 'NONE',  ( -5.250000000000000888, -28.60416666666666430, 3.031088913245533423 ) ) ;
#6770=CARTESIAN_POINT ( 'NONE',  ( 5.250000000000000000, -28.03125000068279604, 0.000000000000000000 ) ) ;
#6777=CARTESIAN_POINT ( 'NONE',  ( -1.975475456537005874E-15, -29.56250000000000000, 5.250000000000000000 ) ) ;
#6779=CARTESIAN_POINT ( 'NONE',  ( 5.249999999999999112, -28.22916666666666430, -3.031088913245534755 ) ) ;
#6780=CARTESIAN_POINT ( 'NONE',  ( 2.033577675846918216E-14, -27.84375000068279959, 5.250000000000000888 ) ) ;
#6781=LINE ( 'NONE', #3255, #4216 ) ;
#6782=CARTESIAN_POINT ( 'NONE',  ( 5.250000000000000000, -27.75000000000000000, 0.000000000000000000 ) ) ;
#6793=EDGE_CURVE ( 'NONE', #7910, #4963, #5106, .T. ) ;
#6795=ORIENTED_EDGE ( 'NONE', *, *, #6392, .F. ) ;
#6800=CARTESIAN_POINT ( 'NONE',  ( 5.114683531250000748, -28.83854166700806587, -2.952963913586932776 ) ) ;
#6802=CARTESIAN_POINT ( 'NONE',  ( -2.625000000000002220, -28.08333333333333215, 4.546633369868302132 ) ) ;
#6803=CARTESIAN_POINT ( 'NONE',  ( 3.616337804771879580E-16, -28.35937500034139447, -5.905927827173866440 ) ) ;
#6807=LINE ( 'NONE', #6709, #2235 ) ;
#6808=CARTESIAN_POINT ( 'NONE',  ( 1.406733260263402174, -27.05133545031536713, 5.249999999999995559 ) ) ;
#6810=CARTESIAN_POINT ( 'NONE',  ( -2.557341765624999042, -28.58854166700806587, -4.429445870380400052 ) ) ;
#6814=CARTESIAN_POINT ( 'NONE',  ( -2.624999999999998668, -28.66666666666666785, -4.546633369868303021 ) ) ;
#6820=CARTESIAN_POINT ( 'NONE',  ( 5.249999999999999112, -29.26041666734946389, -3.031088913245534755 ) ) ;
#6821=CARTESIAN_POINT ( 'NONE',  ( -5.250000000000000000, -28.40625000068279604, -6.429395695523604153E-16 ) ) ;
#6824=EDGE_CURVE ( 'NONE', #1880, #6258, #8643, .T. ) ;
#6826=AXIS2_PLACEMENT_3D ( 'NONE', #5193, #8035, #8638 ) ;
#6829=CARTESIAN_POINT ( 'NONE',  ( 1.406733260263394625, -29.44866454968462932, -5.250000000000000000 ) ) ;
#6830=( BOUNDED_CURVE ( )  B_SPLINE_CURVE ( 2, ( #245, #1596, #7365, #5829, #3097, #1503, #6570, #293, #5875 ),
 .UNSPECIFIED., .F., .T. ) 
 B_SPLINE_CURVE_WITH_KNOTS ( ( 3, 2, 2, 2, 3 ),
 ( 0.1875000000000000000, 0.1944444444444444475, 0.2083333333333333426, 0.2222222222222222099, 0.2291666666666666574 ),
 .UNSPECIFIED. ) 
 CURVE ( )  GEOMETRIC_REPRESENTATION_ITEM ( )  RATIONAL_B_SPLINE_CURVE ( ( 0.9330127018922194093, 0.9330127018922194093, 1.000000000000000000, 0.8660254037844387076, 1.000000000000000000, 0.8660254037844387076, 1.000000000000000000, 0.9330127018922194093, 0.9330127018922194093 ) ) 
 REPRESENTATION_ITEM ( '' )  );
#6831=CARTESIAN_POINT ( 'NONE',  ( 1.185285273922203525E-14, -28.93749999999999645, -5.250000000000000000 ) ) ;
#6834=CARTESIAN_POINT ( 'NONE',  ( -5.114683531250000748, -29.48437500034139802, -6.263680815196995234E-16 ) ) ;
#6835=ORIENTED_EDGE ( 'NONE', *, *, #7462, .T. ) ;
#6840=LINE ( 'NONE', #4053, #7709 ) ;
#6846=VECTOR ( 'NONE', #8597, 1000.000000000000000 ) ;
#6847=DIRECTION ( 'NONE',  ( 0.000000000000000000, 0.000000000000000000, 1.000000000000000000 ) ) ;
#6853=CARTESIAN_POINT ( 'NONE',  ( -5.114683531250000748, -28.73437500034139802, -6.263680815196995234E-16 ) ) ;
#6856=CARTESIAN_POINT ( 'NONE',  ( 5.250000000000000000, -30.00000000000000000, 0.000000000000000000 ) ) ;
#6860=CARTESIAN_POINT ( 'NONE',  ( -1.084901341431563923E-15, -26.92187500034139802, 5.905927827173866440 ) ) ;
#6861=DIRECTION ( 'NONE',  ( 1.000000000000000000, 0.000000000000000000, 0.000000000000000000 ) ) ;
#6862=CARTESIAN_POINT ( 'NONE',  ( 2.557341765624996821, -29.21354166700806587, 4.429445870380401828 ) ) ;
#6865=CARTESIAN_POINT ( 'NONE',  ( -5.250000000000000888, -29.13541666734946389, 3.031088913245533423 ) ) ;
#6866=DIRECTION ( 'NONE',  ( 0.000000000000000000, 1.000000000000000000, 0.000000000000000000 ) ) ;
#6872=CARTESIAN_POINT ( 'NONE',  ( -5.250000000000000000, -28.42708333401612819, -3.031088913245536531 ) ) ;
#6877=CARTESIAN_POINT ( 'NONE',  ( 5.250000000000000000, -29.78125000068279604, 0.000000000000000000 ) ) ;
#6881=VECTOR ( 'NONE', #8983, 1000.000000000000000 ) ;
#6882=CARTESIAN_POINT ( 'NONE',  ( 0.000000000000000000, -9.999999999999998224, 0.000000000000000000 ) ) ;
#6888=CIRCLE ( 'NONE', #8663, 5.250000000000000000 ) ;
#6892=ORIENTED_EDGE ( 'NONE', *, *, #1508, .T. ) ;
#6893=DIRECTION ( 'NONE',  ( 0.000000000000000000, 1.000000000000000000, 0.000000000000000000 ) ) ;
#6894=DIRECTION ( 'NONE',  ( -0.8660254037844402619, 0.4999999999999970579, -0.000000000000000000 ) ) ;
#6902=CARTESIAN_POINT ( 'NONE',  ( 5.114683531249998971, -27.63020833367473017, 2.952963913586936329 ) ) ;
#6904=DIRECTION ( 'NONE',  ( 0.000000000000000000, 1.000000000000000000, 0.000000000000000000 ) ) ;
#6905=CARTESIAN_POINT ( 'NONE',  ( -5.114683531249999859, -27.56770833367473017, -2.952963913586935440 ) ) ;
#6907=CARTESIAN_POINT ( 'NONE',  ( -5.114683531250000748, -26.96354166700806587, 2.952963913586931888 ) ) ;
#6908=CARTESIAN_POINT ( 'NONE',  ( -2.624999999999998668, -28.41666666666666785, -4.546633369868303021 ) ) ;
#6909=CARTESIAN_POINT ( 'NONE',  ( 5.114683531249999859, -28.40104166700806232, -2.952963913586932776 ) ) ;
#6919=CARTESIAN_POINT ( 'NONE',  ( -5.250000000000000888, -27.88541666734946389, 3.031088913245532979 ) ) ;
#6924=FACE_OUTER_BOUND ( 'NONE', #6452, .T. ) ;
#6925=EDGE_CURVE ( 'NONE', #6499, #7888, #1039, .T. ) ;
#6926=CARTESIAN_POINT ( 'NONE',  ( -2.625000000000002220, -28.83333333333333215, 4.546633369868302132 ) ) ;
#6927=CARTESIAN_POINT ( 'NONE',  ( 0.000000000000000000, -30.00000000000000000, 0.000000000000000000 ) ) ;
#6936=LINE ( 'NONE', #9114, #7145 ) ;
#6939=CARTESIAN_POINT ( 'NONE',  ( 5.114683531250000748, -28.08854166700806232, -2.952963913586932776 ) ) ;
#6942=CARTESIAN_POINT ( 'NONE',  ( -5.114683531249999859, -27.06770833367473017, -2.952963913586935440 ) ) ;
#6944=CARTESIAN_POINT ( 'NONE',  ( 2.557341765624996821, -29.21354166700806587, 4.429445870380401828 ) ) ;
#6947=CARTESIAN_POINT ( 'NONE',  ( 5.114683531250000748, -28.92187500034139802, 0.000000000000000000 ) ) ;
#6948=CARTESIAN_POINT ( 'NONE',  ( -5.250000000000000000, -28.90625000068279604, -6.429395695523604153E-16 ) ) ;
#6957=CARTESIAN_POINT ( 'NONE',  ( 2.624999999999996891, -26.82291666734946389, 4.546633369868304797 ) ) ;
#6959=ADVANCED_FACE ( 'NONE', ( #6602 ), #7999, .T. ) ;
#6960=EDGE_LOOP ( 'NONE', ( #2425, #5189, #1698, #4017 ) ) ;
#6963=CARTESIAN_POINT ( 'NONE',  ( 5.250000000000000000, -30.00000000000000000, 0.000000000000000000 ) ) ;
#6970=CARTESIAN_POINT ( 'NONE',  ( -2.557341765624999042, -29.27604166700806232, -4.429445870380400052 ) ) ;
#6977=CARTESIAN_POINT ( 'NONE',  ( -2.625000000000002220, -27.08333333333333570, 4.546633369868302132 ) ) ;
#6982=ORIENTED_EDGE ( 'NONE', *, *, #513, .F. ) ;
#6985=CARTESIAN_POINT ( 'NONE',  ( 5.114683531250000748, -27.35937500034139802, 0.000000000000000000 ) ) ;
#6987=CIRCLE ( 'NONE', #6244, 5.250000000000000000 ) ;
#6988=CARTESIAN_POINT ( 'NONE',  ( -5.114683531250000748, -28.02604166700806587, 2.952963913586931888 ) ) ;
#6989=ADVANCED_FACE ( 'NONE', ( #6036 ), #8046, .F. ) ;
#6990=CARTESIAN_POINT ( 'NONE',  ( -5.114683531250000748, -29.06770833367473017, -2.952963913586935440 ) ) ;
#6993=CARTESIAN_POINT ( 'NONE',  ( -5.114683531250000748, -28.77604166700806587, 2.952963913586931888 ) ) ;
#7004=CARTESIAN_POINT ( 'NONE',  ( 5.114683531249998971, -29.38020833367473017, 2.952963913586936329 ) ) ;
#7006=ORIENTED_EDGE ( 'NONE', *, *, #8391, .T. ) ;
#7009=LINE ( 'NONE', #4987, #4149 ) ;
#7011=CARTESIAN_POINT ( 'NONE',  ( 0.000000000000000000, -30.00000000000000000, 5.250000000000000000 ) ) ;
#7013=CARTESIAN_POINT ( 'NONE',  ( 5.114683531249999859, -28.33854166700806587, -2.952963913586932776 ) ) ;
#7021=CARTESIAN_POINT ( 'NONE',  ( 1.406733260263400176, -28.94866454968462932, -5.249999999999997335 ) ) ;
#7028=CIRCLE ( 'NONE', #5092, 5.750000000000000000 ) ;
#7029=ORIENTED_EDGE ( 'NONE', *, *, #358, .T. ) ;
#7030=CARTESIAN_POINT ( 'NONE',  ( 3.616337804771879580E-16, -28.29687500034139802, -5.905927827173866440 ) ) ;
#7032=CARTESIAN_POINT ( 'NONE',  ( 3.616337804771879580E-16, -27.85937500034139802, -5.905927827173866440 ) ) ;
#7033=ADVANCED_FACE ( 'NONE', ( #7493 ), #560, .T. ) ;
#7036=CARTESIAN_POINT ( 'NONE',  ( 5.114683531249998971, -28.69270833367473017, 2.952963913586936329 ) ) ;
#7038=CARTESIAN_POINT ( 'NONE',  ( -1.084901341431563923E-15, -28.23437500034139802, 5.905927827173866440 ) ) ;
#7041=CIRCLE ( 'NONE', #6594, 4.250000000000000000 ) ;
#7047=CARTESIAN_POINT ( 'NONE',  ( -5.114683531250000748, -29.23437500034139802, -6.263680815196995234E-16 ) ) ;
#7053=EDGE_LOOP ( 'NONE', ( #1806, #4771, #5930, #1744 ) ) ;
#7057=CARTESIAN_POINT ( 'NONE',  ( 5.114683531249998971, -28.88020833367473017, 2.952963913586936329 ) ) ;
#7065=DIRECTION ( 'NONE',  ( 0.000000000000000000, 0.000000000000000000, 1.000000000000000000 ) ) ;
#7066=CARTESIAN_POINT ( 'NONE',  ( -2.625000000000002220, -26.86458333401613174, 4.546633369868302132 ) ) ;
#7067=VERTEX_POINT ( 'NONE', #6232 ) ;
#7071=CARTESIAN_POINT ( 'NONE',  ( 5.114683531249998971, -27.13020833367473372, 2.952963913586936329 ) ) ;
#7074=CARTESIAN_POINT ( 'NONE',  ( -5.250000000000000000, -29.64583333333333215, -3.031088913245536531 ) ) ;
#7077=CARTESIAN_POINT ( 'NONE',  ( 2.557341765624996821, -29.46354166700806232, 4.429445870380401828 ) ) ;
#7078=EDGE_CURVE ( 'NONE', #3105, #5259, #6840, .T. ) ;
#7079=CARTESIAN_POINT ( 'NONE',  ( -2.557341765624999042, -27.08854166700806232, -4.429445870380400052 ) ) ;
#7084=DIRECTION ( 'NONE',  ( 0.000000000000000000, 0.000000000000000000, 1.000000000000000000 ) ) ;
#7085=CARTESIAN_POINT ( 'NONE',  ( 3.616337804771879580E-16, -29.85937500034139802, -5.905927827173866440 ) ) ;
#7089=CARTESIAN_POINT ( 'NONE',  ( 3.712013335537174572E-16, -27.21875000068279604, -6.062177826491070398 ) ) ;
#7101=CARTESIAN_POINT ( 'NONE',  ( 3.616337804771879580E-16, -28.29687500034139802, -5.905927827173866440 ) ) ;
#7104=DIRECTION ( 'NONE',  ( -0.8660254037844402619, -0.4999999999999970579, 0.000000000000000000 ) ) ;
#7112=ORIENTED_EDGE ( 'NONE', *, *, #3553, .F. ) ;
#7119=CARTESIAN_POINT ( 'NONE',  ( 3.712013335537174572E-16, -29.18750000000000000, -6.062177826491070398 ) ) ;
#7122=CARTESIAN_POINT ( 'NONE',  ( 5.114683531249998971, -28.19270833367473017, 2.952963913586936329 ) ) ;
#7125=CARTESIAN_POINT ( 'NONE',  ( 5.114683531250000748, -27.17187500034139802, 0.000000000000000000 ) ) ;
#7129=EDGE_CURVE ( 'NONE', #1374, #7067, #603, .T. ) ;
#7130=CARTESIAN_POINT ( 'NONE',  ( 2.624999999999996891, -29.57291666734946034, 4.546633369868304797 ) ) ;
#7131=CARTESIAN_POINT ( 'NONE',  ( 1.406733260263405061, -28.44866454968462932, -5.249999999999994671 ) ) ;
#7132=CARTESIAN_POINT ( 'NONE',  ( -1.406733260263395735, -29.60491455036742892, 5.250000000000000000 ) ) ;
#7139=CARTESIAN_POINT ( 'NONE',  ( 2.557341765624996821, -29.65104166700806232, 4.429445870380401828 ) ) ;
#7145=VECTOR ( 'NONE', #4655, 1000.000000000000000 ) ;
#7149=CARTESIAN_POINT ( 'NONE',  ( 2.557341765624996821, -28.65104166700806587, 4.429445870380401828 ) ) ;
#7154=CARTESIAN_POINT ( 'NONE',  ( 5.114683531250000748, -29.85937500034139802, 0.000000000000000000 ) ) ;
#7157=DIRECTION ( 'NONE',  ( 0.000000000000000000, 1.000000000000000000, 0.000000000000000000 ) ) ;
#7158=CARTESIAN_POINT ( 'NONE',  ( 2.300847884672513123E-14, -28.21875000068279604, -5.250000000000000000 ) ) ;
#7165=CARTESIAN_POINT ( 'NONE',  ( -2.625000000000002220, -29.83333333333333215, 4.546633369868302132 ) ) ;
#7168=CARTESIAN_POINT ( 'NONE',  ( 5.114683531249998971, -27.94270833367473017, 2.952963913586936329 ) ) ;
#7169=AXIS2_PLACEMENT_3D ( 'NONE', #1177, #6904, #528 ) ;
#7171=CARTESIAN_POINT ( 'NONE',  ( 2.557341765624996821, -27.71354166700806587, 4.429445870380401828 ) ) ;
#7177=CARTESIAN_POINT ( 'NONE',  ( 2.557341765625000818, -29.63020833367473017, -4.429445870380400052 ) ) ;
#7180=VERTEX_POINT ( 'NONE', #8239 ) ;
#7181=CARTESIAN_POINT ( 'NONE',  ( -2.625000000000002220, -28.61458333401612819, 4.546633369868302132 ) ) ;
#7183=CARTESIAN_POINT ( 'NONE',  ( 5.114683531250000748, -27.85937500034139802, 0.000000000000000000 ) ) ;
#7185=AXIS2_PLACEMENT_3D ( 'NONE', #6882, #8917, #7529 ) ;
#7187=DIRECTION ( 'NONE',  ( 0.000000000000000000, 1.000000000000000000, 0.000000000000000000 ) ) ;
#7190=CARTESIAN_POINT ( 'NONE',  ( -1.406733260263395735, -29.07366454968462577, 5.250000000000000000 ) ) ;
#7192=CARTESIAN_POINT ( 'NONE',  ( 2.625000000000000444, -29.23958333401613174, -4.546633369868303021 ) ) ;
#7194=CARTESIAN_POINT ( 'NONE',  ( -2.557341765625002594, -27.44270833367473017, 4.429445870380399164 ) ) ;
#7197=EDGE_CURVE ( 'NONE', #3585, #8002, #1394, .T. ) ;
#7203=CARTESIAN_POINT ( 'NONE',  ( 2.033577675846918216E-14, -27.59375000068279959, 5.250000000000000888 ) ) ;
#7207=VERTEX_POINT ( 'NONE', #7719 ) ;
#7211=CARTESIAN_POINT ( 'NONE',  ( -2.625000000000002220, -29.58333333333333215, 4.546633369868302132 ) ) ;
#7213=CARTESIAN_POINT ( 'NONE',  ( -5.114683531250000748, -28.04687500034139802, -6.263680815196995234E-16 ) ) ;
#7214=CARTESIAN_POINT ( 'NONE',  ( 3.616337804771879580E-16, -27.60937500034139802, -5.905927827173866440 ) ) ;
#7217=CARTESIAN_POINT ( 'NONE',  ( 5.249999999999999112, -28.76041666734946389, -3.031088913245534755 ) ) ;
#7220=ORIENTED_EDGE ( 'NONE', *, *, #4097, .T. ) ;
#7222=CARTESIAN_POINT ( 'NONE',  ( 2.625000000000000444, -26.98958333401612819, -4.546633369868303021 ) ) ;
#7223=CARTESIAN_POINT ( 'NONE',  ( -5.114683531249999859, -29.00520833367473017, -2.952963913586935440 ) ) ;
#7232=CARTESIAN_POINT ( 'NONE',  ( -2.625000000000002220, -29.83333333333333215, 4.546633369868302132 ) ) ;
#7233=CARTESIAN_POINT ( 'NONE',  ( 5.250000000000000000, -29.76041666734946034, -3.031088913245534755 ) ) ;
#7234=ADVANCED_FACE ( 'NONE', ( #2135 ), #1521, .T. ) ;
#7236=CARTESIAN_POINT ( 'NONE',  ( -5.114683531250000748, -27.21354166700806587, 2.952963913586931888 ) ) ;
#7237=FACE_BOUND ( 'NONE', #88, .T. ) ;
#7238=DIRECTION ( 'NONE',  ( 0.000000000000000000, 0.000000000000000000, 1.000000000000000000 ) ) ;
#7240=DIRECTION ( 'NONE',  ( 0.000000000000000000, 0.000000000000000000, 1.000000000000000000 ) ) ;
#7248=ORIENTED_EDGE ( 'NONE', *, *, #7462, .F. ) ;
#7253=ORIENTED_EDGE ( 'NONE', *, *, #8142, .T. ) ;
#7257=CARTESIAN_POINT ( 'NONE',  ( -2.624999999999998668, -29.16666666666666785, -4.546633369868303021 ) ) ;
#7259=CARTESIAN_POINT ( 'NONE',  ( -2.557341765625002594, -27.25520833367473017, 4.429445870380399164 ) ) ;
#7265=CARTESIAN_POINT ( 'NONE',  ( 2.625000000000000444, -28.73958333401612819, -4.546633369868303021 ) ) ;
#7267=CARTESIAN_POINT ( 'NONE',  ( 5.114683531249999859, -29.90104166700806232, -2.952963913586932776 ) ) ;
#7273=CARTESIAN_POINT ( 'NONE',  ( 5.114683531249999859, -28.33854166700806587, -2.952963913586932776 ) ) ;
#7275=VERTEX_POINT ( 'NONE', #7154 ) ;
#7284=CARTESIAN_POINT ( 'NONE',  ( -1.113604000661152470E-15, -29.34375000068279604, 6.062177826491070398 ) ) ;
#7286=CARTESIAN_POINT ( 'NONE',  ( 2.557341765624996821, -27.65104166700806587, 4.429445870380401828 ) ) ;
#7295=CARTESIAN_POINT ( 'NONE',  ( 2.033577675846918216E-14, -27.59375000068279604, 5.250000000000000888 ) ) ;
#7304=EDGE_LOOP ( 'NONE', ( #7307, #7220, #7931, #902, #4983, #4042, #5668, #2080, #1662, #4729, #7112, #3296, #5294, #3680, #1919, #4724, #5516, #7660, #8830, #3031, #274, #132, #1780, #23, #4172, #6215, #1535, #2918 ) ) ;
#7307=ORIENTED_EDGE ( 'NONE', *, *, #5917, .T. ) ;
#7308=CARTESIAN_POINT ( 'NONE',  ( 2.624999999999996891, -27.29166666666666430, 4.546633369868304797 ) ) ;
#7309=CARTESIAN_POINT ( 'NONE',  ( 2.557341765624996821, -28.46354166700806587, 4.429445870380401828 ) ) ;
#7310=EDGE_CURVE ( 'NONE', #8090, #6529, #126, .T. ) ;
#7314=CYLINDRICAL_SURFACE ( 'NONE', #1089, 5.250000000000000000 ) ;
#7317=CARTESIAN_POINT ( 'NONE',  ( -2.557341765624999042, -29.33854166700806232, -4.429445870380400052 ) ) ;
#7320=CARTESIAN_POINT ( 'NONE',  ( -1.975475456537005874E-15, -29.34375000068279249, 5.249999999999999112 ) ) ;
#7321=CARTESIAN_POINT ( 'NONE',  ( 2.557341765624996821, -28.40104166700806587, 4.429445870380401828 ) ) ;
#7322=VERTEX_POINT ( 'NONE', #729 ) ;
#7328=EDGE_LOOP ( 'NONE', ( #2309, #1157, #954, #4462 ) ) ;
#7331=CARTESIAN_POINT ( 'NONE',  ( 5.249999999999999112, -28.80208333401612819, 3.031088913245538308 ) ) ;
#7333=CARTESIAN_POINT ( 'NONE',  ( 2.557341765624996821, -29.71354166700806232, 4.429445870380401828 ) ) ;
#7334=ORIENTED_EDGE ( 'NONE', *, *, #2325, .F. ) ;
#7337=CARTESIAN_POINT ( 'NONE',  ( 5.182341765625000818, -29.96093750017069723, 0.000000000000000000 ) ) ;
#7352=CARTESIAN_POINT ( 'NONE',  ( 5.250000000000000000, -28.49999999999999645, 0.000000000000000000 ) ) ;
#7361=CARTESIAN_POINT ( 'NONE',  ( -2.624999999999998668, -27.44791666734946389, -4.546633369868303021 ) ) ;
#7362=CARTESIAN_POINT ( 'NONE',  ( 5.114683531249998971, -28.94270833367473017, 2.952963913586936329 ) ) ;
#7364=ORIENTED_EDGE ( 'NONE', *, *, #367, .T. ) ;
#7365=CARTESIAN_POINT ( 'NONE',  ( -2.624999999999998668, -29.41666666666666785, -4.546633369868303021 ) ) ;
#7366=CARTESIAN_POINT ( 'NONE',  ( 2.557341765625000818, -28.06770833367473017, -4.429445870380400052 ) ) ;
#7367=ADVANCED_FACE ( 'NONE', ( #6402 ), #7902, .T. ) ;
#7368=ORIENTED_EDGE ( 'NONE', *, *, #8333, .F. ) ;
#7369=LINE ( 'NONE', #5736, #2138 ) ;
#7374=VERTEX_POINT ( 'NONE', #2844 ) ;
#7376=CARTESIAN_POINT ( 'NONE',  ( -5.250000000000000888, -29.63541666734946389, 3.031088913245532979 ) ) ;
#7378=CARTESIAN_POINT ( 'NONE',  ( 3.616337804771879580E-16, -27.29687500034139802, -5.905927827173866440 ) ) ;
#7380=DIRECTION ( 'NONE',  ( 1.000000000000000000, 0.000000000000000000, 0.000000000000000000 ) ) ;
#7382=DIRECTION ( 'NONE',  ( 0.000000000000000000, 1.000000000000000000, 0.000000000000000000 ) ) ;
#7387=DIRECTION ( 'NONE',  ( 0.000000000000000000, 0.000000000000000000, 1.000000000000000000 ) ) ;
#7390=ORIENTED_EDGE ( 'NONE', *, *, #7742, .F. ) ;
#7400=CARTESIAN_POINT ( 'NONE',  ( -5.250000000000000000, -28.37499999999999645, -6.429395695523604153E-16 ) ) ;
#7403=ORIENTED_EDGE ( 'NONE', *, *, #430, .F. ) ;
#7407=CARTESIAN_POINT ( 'NONE',  ( 2.557341765624996821, -28.40104166700806587, 4.429445870380401828 ) ) ;
#7411=CARTESIAN_POINT ( 'NONE',  ( -5.114683531250000748, -28.54687500034139802, -6.263680815196995234E-16 ) ) ;
#7414=CARTESIAN_POINT ( 'NONE',  ( 1.406733260263391960, -29.30133545031537068, 5.250000000000000000 ) ) ;
#7415=CARTESIAN_POINT ( 'NONE',  ( -2.557341765625002594, -26.94270833367473017, 4.429445870380399164 ) ) ;
#7418=EDGE_CURVE ( 'NONE', #3705, #1374, #8085, .T. ) ;
#7427=CARTESIAN_POINT ( 'NONE',  ( -2.624999999999998668, -28.44791666734946389, -4.546633369868303021 ) ) ;
#7429=AXIS2_PLACEMENT_3D ( 'NONE', #5054, #2322, #2229 ) ;
#7439=VECTOR ( 'NONE', #9070, 1000.000000000000000 ) ;
#7440=CARTESIAN_POINT ( 'NONE',  ( 2.557341765625000818, -29.56770833367473017, -4.429445870380400052 ) ) ;
#7450=CARTESIAN_POINT ( 'NONE',  ( 3.712013335537174572E-16, -27.43750000000000000, -6.062177826491070398 ) ) ;
#7454=( NAMED_UNIT ( * ) SI_UNIT ( $, .STERADIAN. ) SOLID_ANGLE_UNIT ( ) );
#7457=CARTESIAN_POINT ( 'NONE',  ( -5.114683531250000748, -29.23437500034139802, -6.263680815196995234E-16 ) ) ;
#7459=CARTESIAN_POINT ( 'NONE',  ( 2.300847884672513123E-14, -27.21875000068279959, -5.250000000000000000 ) ) ;
#7460=CARTESIAN_POINT ( 'NONE',  ( 5.114683531249999859, -28.65104166700806587, -2.952963913586932776 ) ) ;
#7462=EDGE_CURVE ( 'NONE', #1378, #4147, #5015, .T. ) ;
#7463=CARTESIAN_POINT ( 'NONE',  ( -2.324088772396477476E-15, -29.46875000068279959, -5.250000000000000000 ) ) ;
#7464=CARTESIAN_POINT ( 'NONE',  ( 5.114683531250000748, -26.85937500034139802, 0.000000000000000000 ) ) ;
#7471=VERTEX_POINT ( 'NONE', #8731 ) ;
#7473=CARTESIAN_POINT ( 'NONE',  ( -2.625000000000002220, -27.86458333401612819, 4.546633369868302132 ) ) ;
#7476=ORIENTED_EDGE ( 'NONE', *, *, #367, .F. ) ;
#7479=DIRECTION ( 'NONE',  ( 0.000000000000000000, 1.000000000000000000, 0.000000000000000000 ) ) ;
#7483=CARTESIAN_POINT ( 'NONE',  ( -5.249999999999999112, -28.89583333333333215, -3.031088913245536975 ) ) ;
#7485=CARTESIAN_POINT ( 'NONE',  ( 2.625000000000000444, -27.98958333401612819, -4.546633369868303021 ) ) ;
#7488=CARTESIAN_POINT ( 'NONE',  ( 5.249999999999999112, -27.72916666666666430, -3.031088913245534755 ) ) ;
#7493=FACE_OUTER_BOUND ( 'NONE', #1453, .T. ) ;
#7497=CARTESIAN_POINT ( 'NONE',  ( 5.250000000000000000, -27.99999999999999645, 0.000000000000000000 ) ) ;
#7500=EDGE_LOOP ( 'NONE', ( #2457, #6556, #7521, #1193 ) ) ;
#7503=CARTESIAN_POINT ( 'NONE',  ( 5.114683531250000748, -28.33854166700806587, -2.952963913586932776 ) ) ;
#7506=CYLINDRICAL_SURFACE ( 'NONE', #7169, 5.250000000000000000 ) ;
#7507=CARTESIAN_POINT ( 'NONE',  ( -1.084901341431563923E-15, -28.73437500034139802, 5.905927827173866440 ) ) ;
#7509=CYLINDRICAL_SURFACE ( 'NONE', #2548, 5.250000000000000000 ) ;
#7511=DIRECTION ( 'NONE',  ( -0.000000000000000000, -1.000000000000000000, -0.000000000000000000 ) ) ;
#7517=ORIENTED_EDGE ( 'NONE', *, *, #2193, .T. ) ;
#7519=CARTESIAN_POINT ( 'NONE',  ( -5.250000000000000000, -28.15625000068279604, -6.429395695523604153E-16 ) ) ;
#7521=ORIENTED_EDGE ( 'NONE', *, *, #4460, .F. ) ;
#7524=CARTESIAN_POINT ( 'NONE',  ( 0.000000000000000000, 75.00000000000000000, 0.000000000000000000 ) ) ;
#7525=EDGE_CURVE ( 'NONE', #8002, #1439, #5239, .T. ) ;
#7527=CARTESIAN_POINT ( 'NONE',  ( 2.625000000000000444, -28.20833333333333215, -4.546633369868303021 ) ) ;
#7529=DIRECTION ( 'NONE',  ( 0.000000000000000000, 0.000000000000000000, 1.000000000000000000 ) ) ;
#7535=CARTESIAN_POINT ( 'NONE',  ( 0.000000000000000000, -30.00000000000000000, 0.000000000000000000 ) ) ;
#7540=CARTESIAN_POINT ( 'NONE',  ( 6.429395695523604153E-16, -30.00000000000000000, -5.250000000000000000 ) ) ;
#7548=CARTESIAN_POINT ( 'NONE',  ( -1.084901341431563726E-15, -28.67187500034139802, 5.905927827173866440 ) ) ;
#7550=CARTESIAN_POINT ( 'NONE',  ( -1.406733260263385521, -28.07366454968462932, 5.250000000000006217 ) ) ;
#7551=CARTESIAN_POINT ( 'NONE',  ( 2.557341765624996821, -27.46354166700806587, 4.429445870380401828 ) ) ;
#7553=DIRECTION ( 'NONE',  ( 0.000000000000000000, 1.000000000000000000, 0.000000000000000000 ) ) ;
#7555=CARTESIAN_POINT ( 'NONE',  ( -5.114683531250000748, -27.46354166700806232, 2.952963913586931888 ) ) ;
#7557=CARTESIAN_POINT ( 'NONE',  ( -5.114683531249999859, -28.81770833367473017, -2.952963913586935440 ) ) ;
#7560=ADVANCED_FACE ( 'NONE', ( #1615 ), #1060, .F. ) ;
#7561=CARTESIAN_POINT ( 'NONE',  ( -5.249999999999999112, -28.64583333333332860, -3.031088913245536975 ) ) ;
#7562=CARTESIAN_POINT ( 'NONE',  ( 6.429395695523604153E-16, -30.00000000000000000, -5.250000000000000000 ) ) ;
#7568=CARTESIAN_POINT ( 'NONE',  ( -2.625000000000002220, -27.36458333401612819, 4.546633369868302132 ) ) ;
#7576=EDGE_CURVE ( 'NONE', #803, #7933, #2409, .T. ) ;
#7577=CARTESIAN_POINT ( 'NONE',  ( -5.250000000000000888, -28.85416666666667140, 3.031088913245533423 ) ) ;
#7578=LINE ( 'NONE', #6028, #2879 ) ;
#7580=CARTESIAN_POINT ( 'NONE',  ( 2.300847884672513123E-14, -27.96875000068279959, -5.250000000000000000 ) ) ;
#7581=CARTESIAN_POINT ( 'NONE',  ( -1.975475456537005874E-15, -27.34375000068279249, 5.249999999999999112 ) ) ;
#7590=ORIENTED_EDGE ( 'NONE', *, *, #358, .F. ) ;
#7591=CARTESIAN_POINT ( 'NONE',  ( 6.429395695523604153E-16, -30.00000000000000000, -5.250000000000000000 ) ) ;
#7599=CARTESIAN_POINT ( 'NONE',  ( 5.114683531250000748, -27.85937500034139802, 0.000000000000000000 ) ) ;
#7602=CARTESIAN_POINT ( 'NONE',  ( -5.114683531250000748, -27.77604166700806587, 2.952963913586931888 ) ) ;
#7603=FACE_OUTER_BOUND ( 'NONE', #8980, .T. ) ;
#7604=CARTESIAN_POINT ( 'NONE',  ( 6.429395695523604153E-16, -30.00000000000000000, -5.250000000000000000 ) ) ;
#7605=CYLINDRICAL_SURFACE ( 'NONE', #6525, 4.250000000000000000 ) ;
#7606=EDGE_CURVE ( 'NONE', #7933, #7374, #5625, .T. ) ;
#7607=CARTESIAN_POINT ( 'NONE',  ( 5.114683531250000748, -29.17187500034139802, 0.000000000000000000 ) ) ;
#7611=CARTESIAN_POINT ( 'NONE',  ( 0.000000000000000000, -30.00000000000000000, 0.000000000000000000 ) ) ;
#7616=CARTESIAN_POINT ( 'NONE',  ( 5.250000000000000000, -29.28125000068279604, 0.000000000000000000 ) ) ;
#7617=CARTESIAN_POINT ( 'NONE',  ( -5.250000000000000888, -28.13541666734947100, 3.031088913245532979 ) ) ;
#7622=DIRECTION ( 'NONE',  ( 0.000000000000000000, 0.000000000000000000, 1.000000000000000000 ) ) ;
#7623=CARTESIAN_POINT ( 'NONE',  ( 1.406733260263405061, -28.19866454968462577, -5.249999999999994671 ) ) ;
#7626=CARTESIAN_POINT ( 'NONE',  ( -2.557341765625002594, -29.69270833367473017, 4.429445870380399164 ) ) ;
#7627=DIRECTION ( 'NONE',  ( 0.000000000000000000, 1.000000000000000000, 0.000000000000000000 ) ) ;
#7632=AXIS2_PLACEMENT_3D ( 'NONE', #9012, #7627, #1256 ) ;
#7637=AXIS2_PLACEMENT_3D ( 'NONE', #5937, #5797, #3807 ) ;
#7641=CARTESIAN_POINT ( 'NONE',  ( 5.114683531249998971, -28.13020833367473017, 2.952963913586936329 ) ) ;
#7644=CARTESIAN_POINT ( 'NONE',  ( -5.114683531250000748, -27.27604166700806232, 2.952963913586931888 ) ) ;
#7646=EDGE_CURVE ( 'NONE', #8929, #5643, #5325, .T. ) ;
#7647=CARTESIAN_POINT ( 'NONE',  ( -2.557341765624999042, -29.33854166700806232, -4.429445870380400052 ) ) ;
#7649=CARTESIAN_POINT ( 'NONE',  ( -1.406733260263382856, -28.42633545031537068, -5.250000000000006217 ) ) ;
#7650=CARTESIAN_POINT ( 'NONE',  ( 5.114683531249998971, -28.69270833367473017, 2.952963913586936329 ) ) ;
#7656=DIRECTION ( 'NONE',  ( 1.000000000000000000, 0.000000000000000000, 0.000000000000000000 ) ) ;
#7660=ORIENTED_EDGE ( 'NONE', *, *, #8818, .F. ) ;
#7662=CARTESIAN_POINT ( 'NONE',  ( -1.113604000661152470E-15, -26.84375000068279959, 6.062177826491070398 ) ) ;
#7668=PLANE ( 'NONE',  #4473 ) ;
#7671=CARTESIAN_POINT ( 'NONE',  ( 3.616337804771879580E-16, -28.04687500034139802, -5.905927827173866440 ) ) ;
#7680=CARTESIAN_POINT ( 'NONE',  ( -5.250000000000000888, -27.13541666734946389, 3.031088913245533423 ) ) ;
#7684=CARTESIAN_POINT ( 'NONE',  ( 2.557341765625000818, -27.81770833367473017, -4.429445870380400052 ) ) ;
#7686=CARTESIAN_POINT ( 'NONE',  ( -5.114683531250000748, -27.04687500034139802, -6.263680815196995234E-16 ) ) ;
#7689=CARTESIAN_POINT ( 'NONE',  ( 5.114683531249998971, -29.44270833367473372, 2.952963913586936329 ) ) ;
#7690=DIRECTION ( 'NONE',  ( 0.000000000000000000, 1.000000000000000000, 0.000000000000000000 ) ) ;
#7691=CARTESIAN_POINT ( 'NONE',  ( 5.114683531249998971, -29.69270833367473017, 2.952963913586936329 ) ) ;
#7699=ORIENTED_EDGE ( 'NONE', *, *, #4628, .T. ) ;
#7701=CARTESIAN_POINT ( 'NONE',  ( 5.114683531250000748, -29.35937500034139802, 0.000000000000000000 ) ) ;
#7705=VERTEX_POINT ( 'NONE', #1109 ) ;
#7709=VECTOR ( 'NONE', #8969, 1000.000000000000000 ) ;
#7712=ADVANCED_FACE ( 'NONE', ( #8958 ), #5523, .T. ) ;
#7715=CARTESIAN_POINT ( 'NONE',  ( 2.557341765625000818, -28.31770833367473017, -4.429445870380400052 ) ) ;
#7717=EDGE_CURVE ( 'NONE', #6430, #5221, #3996, .T. ) ;
#7719=CARTESIAN_POINT ( 'NONE',  ( 6.972266317189433020E-16, -29.43750000000000000, -5.249999999999999112 ) ) ;
#7724=CARTESIAN_POINT ( 'NONE',  ( 5.250000000000000000, -27.25000000000000000, 0.000000000000000000 ) ) ;
#7725=CARTESIAN_POINT ( 'NONE',  ( -2.625000000000002220, -27.86458333401612819, 4.546633369868302132 ) ) ;
#7727=EDGE_LOOP ( 'NONE', ( #8666, #6603, #5918, #2922, #3537, #4625, #1421, #960 ) ) ;
#7732=CARTESIAN_POINT ( 'NONE',  ( -2.557341765624999042, -28.27604166700806587, -4.429445870380400052 ) ) ;
#7735=CARTESIAN_POINT ( 'NONE',  ( 5.114683531250000748, -26.92187500034139802, 0.000000000000000000 ) ) ;
#7737=CARTESIAN_POINT ( 'NONE',  ( 2.557341765624996821, -28.96354166700806587, 4.429445870380401828 ) ) ;
#7740=CARTESIAN_POINT ( 'NONE',  ( -5.114683531250000748, -27.27604166700806232, 2.952963913586931888 ) ) ;
#7741=CARTESIAN_POINT ( 'NONE',  ( -5.249999999999999112, -29.64583333333333215, -3.031088913245536975 ) ) ;
#7742=EDGE_CURVE ( 'NONE', #6258, #7207, #2661, .T. ) ;
#7751=CARTESIAN_POINT ( 'NONE',  ( 3.616337804771879580E-16, -29.79687500034140157, -5.905927827173866440 ) ) ;
#7759=ADVANCED_FACE ( 'NONE', ( #6924 ), #3251, .T. ) ;
#7760=CARTESIAN_POINT ( 'NONE',  ( 3.616337804771879580E-16, -28.79687500034139802, -5.905927827173866440 ) ) ;
#7769=DIRECTION ( 'NONE',  ( 0.000000000000000000, -0.000000000000000000, 1.000000000000000000 ) ) ;
#7771=DIRECTION ( 'NONE',  ( 0.000000000000000000, 0.000000000000000000, 1.000000000000000000 ) ) ;
#7776=AXIS2_PLACEMENT_3D ( 'NONE', #8438, #2064, #4249 ) ;
#7777=CARTESIAN_POINT ( 'NONE',  ( 5.114683531250000748, -28.10937500034139447, 0.000000000000000000 ) ) ;
#7779=CARTESIAN_POINT ( 'NONE',  ( 5.249999999999999112, -29.77083333333333570, 3.031088913245538308 ) ) ;
#7784=CARTESIAN_POINT ( 'NONE',  ( -5.114683531250001636, -29.27604166700806232, 2.952963913586931444 ) ) ;
#7787=CARTESIAN_POINT ( 'NONE',  ( 2.557341765625000818, -27.13020833367473017, -4.429445870380400052 ) ) ;
#7797=ORIENTED_EDGE ( 'NONE', *, *, #8371, .F. ) ;
#7799=CARTESIAN_POINT ( 'NONE',  ( -5.250000000000000000, -27.15625000068279604, -6.429395695523604153E-16 ) ) ;
#7800=VERTEX_POINT ( 'NONE', #1810 ) ;
#7803=DIRECTION ( 'NONE',  ( 0.000000000000000000, -0.000000000000000000, 1.000000000000000000 ) ) ;
#7808=CARTESIAN_POINT ( 'NONE',  ( 2.557341765625000818, -28.56770833367473017, -4.429445870380400052 ) ) ;
#7810=CARTESIAN_POINT ( 'NONE',  ( 1.406733260263391960, -29.08258545099816317, 5.250000000000000000 ) ) ;
#7815=CARTESIAN_POINT ( 'NONE',  ( 6.972266317189433020E-16, -27.18750000000000000, -5.250000000000000000 ) ) ;
#7817=EDGE_CURVE ( 'NONE', #4147, #1378, #5767, .T. ) ;
#7818=EDGE_LOOP ( 'NONE', ( #6347, #2496, #5648, #1947 ) ) ;
#7824=CARTESIAN_POINT ( 'NONE',  ( 5.250000000000000000, -28.99999999999999645, 0.000000000000000000 ) ) ;
#7826=CARTESIAN_POINT ( 'NONE',  ( -5.114683531250000748, -29.54687500034139802, -6.263680815196995234E-16 ) ) ;
#7827=CARTESIAN_POINT ( 'NONE',  ( -2.557341765625002594, -28.00520833367473017, 4.429445870380399164 ) ) ;
#7830=FACE_OUTER_BOUND ( 'NONE', #8721, .T. ) ;
#7832=CARTESIAN_POINT ( 'NONE',  ( 1.406733260263397289, -28.55133545031537068, 5.249999999999997335 ) ) ;
#7833=CARTESIAN_POINT ( 'NONE',  ( -5.249999999999999112, -29.67708333401613530, -3.031088913245536975 ) ) ;
#7834=( BOUNDED_CURVE ( )  B_SPLINE_CURVE ( 2, ( #3222, #8016, #1502, #1647, #4345, #1076, #7181, #3648, #6278 ),
 .UNSPECIFIED., .F., .T. ) 
 B_SPLINE_CURVE_WITH_KNOTS ( ( 3, 2, 2, 2, 3 ),
 ( 0.3541666666666666297, 0.3611111111111111049, 0.3750000000000000000, 0.3888888888888888951, 0.3958333333333333703 ),
 .UNSPECIFIED. ) 
 CURVE ( )  GEOMETRIC_REPRESENTATION_ITEM ( )  RATIONAL_B_SPLINE_CURVE ( ( 0.9330127018922194093, 0.9330127018922190762, 1.000000000000000000, 0.8660254037844387076, 1.000000000000000000, 0.8660254037844387076, 1.000000000000000000, 0.9330127018922190762, 0.9330127018922194093 ) ) 
 REPRESENTATION_ITEM ( '' )  );
#7838=CARTESIAN_POINT ( 'NONE',  ( -1.084901341431563923E-15, -29.42187500034139447, 5.905927827173866440 ) ) ;
#7847=CARTESIAN_POINT ( 'NONE',  ( 2.300847884672513123E-14, -27.96875000068279959, -5.250000000000000000 ) ) ;
#7850=CARTESIAN_POINT ( 'NONE',  ( 5.114683531250000748, -28.10937500034139447, 0.000000000000000000 ) ) ;
#7856=EDGE_CURVE ( 'NONE', #3802, #2565, #3904, .T. ) ;
#7859=CARTESIAN_POINT ( 'NONE',  ( -5.250000000000000000, -27.65625000068279959, -6.429395695523604153E-16 ) ) ;
#7867=CARTESIAN_POINT ( 'NONE',  ( -1.113604000661152470E-15, -29.31249999999999645, 6.062177826491070398 ) ) ;
#7869=CARTESIAN_POINT ( 'NONE',  ( -5.114683531250000748, -28.29687500034139447, -6.263680815196995234E-16 ) ) ;
#7871=CLOSED_SHELL ( 'NONE', ( #9140, #1043, #8, #7560, #6989, #8288, #5068, #8606, #4588, #7712, #1761, #5595, #7367, #1567, #1838, #4068, #6385, #4688, #7033, #6959, #2593, #4072, #5331, #2712, #6406, #6107, #3591, #6128, #826, #7759, #4637, #5496, #4942, #2140, #5135, #419, #7234, #2048, #2182, #4161, #8101, #1953, #4237, #1110, #553, #5800, #1468 ) ) ;
#7872=( NAMED_UNIT ( * ) PLANE_ANGLE_UNIT ( ) SI_UNIT ( $, .RADIAN. ) );
#7873=CARTESIAN_POINT ( 'NONE',  ( 2.557341765624996821, -27.46354166700806587, 4.429445870380401828 ) ) ;
#7874=CIRCLE ( 'NONE', #8026, 5.250000000000000000 ) ;
#7876=CARTESIAN_POINT ( 'NONE',  ( 0.000000000000000000, -9.999999999999998224, 0.000000000000000000 ) ) ;
#7877=DIRECTION ( 'NONE',  ( 0.000000000000000000, -1.000000000000000000, 0.000000000000000000 ) ) ;
#7884=AXIS2_PLACEMENT_3D ( 'NONE', #3628, #7157, #6494 ) ;
#7885=CARTESIAN_POINT ( 'NONE',  ( 2.557341765624996821, -27.90104166700806587, 4.429445870380401828 ) ) ;
#7887=ORIENTED_EDGE ( 'NONE', *, *, #7197, .T. ) ;
#7888=VERTEX_POINT ( 'NONE', #4823 ) ;
#7889=DIRECTION ( 'NONE',  ( 0.000000000000000000, 1.000000000000000000, 0.000000000000000000 ) ) ;
#7898=CARTESIAN_POINT ( 'NONE',  ( 5.114683531249999859, -27.08854166700806232, -2.952963913586932776 ) ) ;
#7902=CYLINDRICAL_SURFACE ( 'NONE', #424, 5.250000000000000000 ) ;
#7906=CARTESIAN_POINT ( 'NONE',  ( -2.624999999999998668, -27.91666666666666430, -4.546633369868303021 ) ) ;
#7910=VERTEX_POINT ( 'NONE', #1511 ) ;
#7914=CARTESIAN_POINT ( 'NONE',  ( 5.250000000000000000, -29.50000000000000000, 0.000000000000000000 ) ) ;
#7916=CARTESIAN_POINT ( 'NONE',  ( -2.557341765624999042, -27.58854166700806587, -4.429445870380400052 ) ) ;
#7918=CARTESIAN_POINT ( 'NONE',  ( 2.557341765625000818, -27.88020833367473017, -4.429445870380400052 ) ) ;
#7919=CARTESIAN_POINT ( 'NONE',  ( -2.557341765625002594, -29.69270833367473017, 4.429445870380399164 ) ) ;
#7924=CARTESIAN_POINT ( 'NONE',  ( 5.114683531250000748, -29.42187500034139802, 0.000000000000000000 ) ) ;
#7925=CYLINDRICAL_SURFACE ( 'NONE', #1991, 2.750000000000000000 ) ;
#7926=EDGE_CURVE ( 'NONE', #784, #5221, #1346, .T. ) ;
#7930=CARTESIAN_POINT ( 'NONE',  ( 5.114683531249998971, -28.38020833367473372, 2.952963913586936329 ) ) ;
#7931=ORIENTED_EDGE ( 'NONE', *, *, #7418, .T. ) ;
#7933=VERTEX_POINT ( 'NONE', #6963 ) ;
#7943=CARTESIAN_POINT ( 'NONE',  ( -5.114683531250000748, -27.48437500034139802, -6.263680815196995234E-16 ) ) ;
#7960=CARTESIAN_POINT ( 'NONE',  ( 2.624999999999996891, -29.54166666666666430, 4.546633369868304797 ) ) ;
#7961=CARTESIAN_POINT ( 'NONE',  ( -2.557341765625002594, -28.25520833367473017, 4.429445870380399164 ) ) ;
#7963=CARTESIAN_POINT ( 'NONE',  ( 5.114683531250000748, -26.89062500034139802, 0.000000000000000000 ) ) ;
#7968=CARTESIAN_POINT ( 'NONE',  ( -1.406733260263393293, -29.70758545099816317, -5.250000000000000000 ) ) ;
#7969=FACE_OUTER_BOUND ( 'NONE', #3177, .T. ) ;
#7972=CARTESIAN_POINT ( 'NONE',  ( -1.084901341431563923E-15, -28.92187500034139447, 5.905927827173866440 ) ) ;
#7973=ORIENTED_EDGE ( 'NONE', *, *, #7856, .T. ) ;
#7982=CARTESIAN_POINT ( 'NONE',  ( 5.114683531249998971, -27.63020833367473017, 2.952963913586936329 ) ) ;
#7983=LINE ( 'NONE', #4407, #6726 ) ;
#7993=( BOUNDED_CURVE ( )  B_SPLINE_CURVE ( 2, ( #3329, #6808, #3373, #8938, #1934 ),
 .UNSPECIFIED., .F., .F. ) 
 B_SPLINE_CURVE_WITH_KNOTS ( ( 3, 2, 3 ),
 ( 0.9791666666666667407, 0.9861111111111111605, 1.000000000000000000 ),
 .UNSPECIFIED. ) 
 CURVE ( )  GEOMETRIC_REPRESENTATION_ITEM ( )  RATIONAL_B_SPLINE_CURVE ( ( 0.9330127018922192983, 0.9330127018922198534, 1.000000000000000000, 0.8660254037844387076, 1.000000000000000000 ) ) 
 REPRESENTATION_ITEM ( '' )  );
#7999=CYLINDRICAL_SURFACE ( 'NONE', #5176, 5.250000000000000000 ) ;
#8002=VERTEX_POINT ( 'NONE', #6346 ) ;
#8003=CARTESIAN_POINT ( 'NONE',  ( -2.625000000000002220, -27.33333333333333215, 4.546633369868302132 ) ) ;
#8006=CARTESIAN_POINT ( 'NONE',  ( 5.114683531249998971, -28.44270833367473017, 2.952963913586936329 ) ) ;
#8007=CARTESIAN_POINT ( 'NONE',  ( -1.406733260263394847, -29.45758545099816317, -5.250000000000000000 ) ) ;
#8011=CARTESIAN_POINT ( 'NONE',  ( 1.406733260263394625, -28.69866454968462577, -5.250000000000000000 ) ) ;
#8012=CARTESIAN_POINT ( 'NONE',  ( 5.114683531250000748, -28.67187500034139802, 0.000000000000000000 ) ) ;
#8013=CARTESIAN_POINT ( 'NONE',  ( 1.406733260263405061, -28.22991455036742181, -5.249999999999994671 ) ) ;
#8015=AXIS2_PLACEMENT_3D ( 'NONE', #2908, #4811, #7656 ) ;
#8016=CARTESIAN_POINT ( 'NONE',  ( -1.406733260263387963, -28.70758545099816672, -5.250000000000001776 ) ) ;
#8018=CARTESIAN_POINT ( 'NONE',  ( 5.114683531250000748, -28.85937500034139802, 0.000000000000000000 ) ) ;
#8020=ORIENTED_EDGE ( 'NONE', *, *, #8892, .F. ) ;
#8026=AXIS2_PLACEMENT_3D ( 'NONE', #130, #3670, #7771 ) ;
#8027=CYLINDRICAL_SURFACE ( 'NONE', #2079, 5.250000000000000000 ) ;
#8028=CARTESIAN_POINT ( 'NONE',  ( 2.624999999999996891, -28.82291666734946389, 4.546633369868304797 ) ) ;
#8030=CARTESIAN_POINT ( 'NONE',  ( -5.114683531250000748, -26.96354166700806587, 2.952963913586931888 ) ) ;
#8035=DIRECTION ( 'NONE',  ( 0.000000000000000000, 1.000000000000000000, 0.000000000000000000 ) ) ;
#8046=CYLINDRICAL_SURFACE ( 'NONE', #8312, 4.250000000000000000 ) ;
#8051=CARTESIAN_POINT ( 'NONE',  ( 5.250000000000000000, -28.47916666666666785, -3.031088913245534755 ) ) ;
#8053=( BOUNDED_CURVE ( )  B_SPLINE_CURVE ( 2, ( #8158, #1133, #5307, #2483, #3973, #5963, #3230, #8801, #333 ),
 .UNSPECIFIED., .F., .F. ) 
 B_SPLINE_CURVE_WITH_KNOTS ( ( 3, 2, 2, 2, 3 ),
 ( 0.3958333333333333703, 0.4027777777777777901, 0.4166666666666666852, 0.4305555555555555802, 0.4375000000000000000 ),
 .UNSPECIFIED. ) 
 CURVE ( )  GEOMETRIC_REPRESENTATION_ITEM ( )  RATIONAL_B_SPLINE_CURVE ( ( 0.9330127018922194093, 0.9330127018922196314, 1.000000000000000000, 0.8660254037844387076, 1.000000000000000000, 0.8660254037844387076, 1.000000000000000000, 0.9330127018922194093, 0.9330127018922194093 ) ) 
 REPRESENTATION_ITEM ( '' )  );
#8054=CARTESIAN_POINT ( 'NONE',  ( -5.114683531250001636, -27.52604166700806587, 2.952963913586931444 ) ) ;
#8055=SURFACE_STYLE_FILL_AREA ( #937 ) ;
#8057=CARTESIAN_POINT ( 'NONE',  ( 0.000000000000000000, -9.000000000000001776, 0.000000000000000000 ) ) ;
#8061=CARTESIAN_POINT ( 'NONE',  ( -5.114683531249999859, -28.81770833367473017, -2.952963913586935440 ) ) ;
#8062=EDGE_LOOP ( 'NONE', ( #8630, #5400, #8096, #8290 ) ) ;
#8066=CARTESIAN_POINT ( 'NONE',  ( -1.084901341431563923E-15, -28.17187500034139447, 5.905927827173866440 ) ) ;
#8067=EDGE_CURVE ( 'NONE', #3693, #2716, #7009, .T. ) ;
#8068=EDGE_LOOP ( 'NONE', ( #8407, #5762 ) ) ;
#8069=CARTESIAN_POINT ( 'NONE',  ( 5.250000000000000000, -26.78125000068279604, 0.000000000000000000 ) ) ;
#8073=CARTESIAN_POINT ( 'NONE',  ( -5.249999999999999112, -29.14583333333333925, -3.031088913245536975 ) ) ;
#8075=ORIENTED_EDGE ( 'NONE', *, *, #5081, .T. ) ;
#8076=CARTESIAN_POINT ( 'NONE',  ( -5.250000000000000888, -29.85416666666666430, 3.031088913245533423 ) ) ;
#8077=CARTESIAN_POINT ( 'NONE',  ( 5.250000000000000000, -28.76041666734946389, -3.031088913245534755 ) ) ;
#8081=CARTESIAN_POINT ( 'NONE',  ( -2.557341765624999042, -27.52604166700806587, -4.429445870380400052 ) ) ;
#8082=ORIENTED_EDGE ( 'NONE', *, *, #74, .F. ) ;
#8083=CYLINDRICAL_SURFACE ( 'NONE', #7637, 5.250000000000000000 ) ;
#8085=LINE ( 'NONE', #3116, #1611 ) ;
#8090=VERTEX_POINT ( 'NONE', #3566 ) ;
#8096=ORIENTED_EDGE ( 'NONE', *, *, #3103, .F. ) ;
#8100=CARTESIAN_POINT ( 'NONE',  ( -5.250000000000000888, -27.60416666666666785, 3.031088913245532979 ) ) ;
#8101=ADVANCED_FACE ( 'NONE', ( #1461, #4308 ), #676, .T. ) ;
#8103=ORIENTED_EDGE ( 'NONE', *, *, #4907, .T. ) ;
#8105=ORIENTED_EDGE ( 'NONE', *, *, #7576, .F. ) ;
#8106=CARTESIAN_POINT ( 'NONE',  ( -5.114683531250000748, -28.50520833367472662, -2.952963913586935440 ) ) ;
#8109=CARTESIAN_POINT ( 'NONE',  ( -2.624999999999998668, -28.16666666666666785, -4.546633369868303021 ) ) ;
#8110=CARTESIAN_POINT ( 'NONE',  ( 5.114683531249999859, -29.15104166700806232, -2.952963913586932776 ) ) ;
#8111=CARTESIAN_POINT ( 'NONE',  ( 0.000000000000000000, -9.999999999999998224, 0.000000000000000000 ) ) ;
#8114=CARTESIAN_POINT ( 'NONE',  ( 2.624999999999996891, -29.29166666666666785, 4.546633369868304797 ) ) ;
#8115=CARTESIAN_POINT ( 'NONE',  ( 3.616337804771879580E-16, -27.04687500034139802, -5.905927827173866440 ) ) ;
#8116=VERTEX_POINT ( 'NONE', #3610 ) ;
#8123=EDGE_LOOP ( 'NONE', ( #1532, #2828 ) ) ;
#8125=CARTESIAN_POINT ( 'NONE',  ( 5.249999999999999112, -29.55208333401613885, 3.031088913245538308 ) ) ;
#8132=CARTESIAN_POINT ( 'NONE',  ( 0.000000000000000000, 75.00000000000000000, 0.000000000000000000 ) ) ;
#8133=( BOUNDED_SURFACE ( )  B_SPLINE_SURFACE ( 1, 2, ( 
 ( #4295, #7267, #2295, #7085, #6377, #5120, #6468, #801, #8571, #6566, #4341, #4432, #199, #2200, #7177, #103, #5773, #17, #5071, #3599, #8616, #2247, #2865, #754, #7924, #4482, #2439, #8758, #7317, #5965, #8935, #1836, #1691, #3832, #288, #2533, #3232, #8110, #3975, #2389, #1087, #5170, #986, #428, #4575, #6053, #3929, #7362, #5265, #3884, #6757, #383, #5219, #8061, #1739, #3145, #3276, #7507, #8891, #6105, #8012, #7460, #5357, #6658, #8802, #4531, #7411, #8205, #1034, #6706, #1135, #1643, #4668, #943, #335, #6803, #3188, #3791, #6615, #242, #5916, #3093, #6009, #8848, #2485, #5308, #8160, #1789, #4622, #4066, #4197, #6988, #2719, #2016, #3415, #4758, #3325, #8347, #8430, #7032, #1972, #9121, #479, #7602, #1887, #9029, #6156, #4712, #3370, #6324, #2058, #8297, #1226, #6905, #2766, #1310, #4883, #5586, #7551, #529, #2584, #6201, #615, #4152, #3501, #4841, #5544, #7644, #2674, #3456, #8984, #1358, #659, #2633, #5404, #5452, #4021, #6942, #7686, #8254, #1178, #1930, #6285, #8389, #7735 ),
 ( #6856, #5501, #4801, #1272, #4110, #571, #6245, #9077, #7165, #744, #8479, #7779, #2285, #697, #2189, #4242, #8521, #7074, #4286, #5061, #7211, #2900, #7960, #6367, #7914, #9160, #4970, #4425, #8561, #836, #1536, #2149, #6413, #7867, #4379, #3681, #3542, #6, #5718, #7119, #7257, #5111, #6503, #884, #3734, #2237, #140, #1440, #7824, #2857, #3589, #2992, #52, #5673, #1584, #2809, #8653, #5629, #5011, #5815, #1489, #2103, #4926, #1401, #4333, #792, #3637, #6459, #92, #2942, #5763, #8605, #7352, #8051, #8195, #1776, #6695, #5999, #7400, #8746, #2426, #5255, #4565, #5210, #4523, #5861, #5345, #978, #6743, #1632, #3042, #3132, #5298, #324, #1023, #3824, #7497, #1823, #2519, #373, #4612, #3085, #278, #8838, #8878, #932, #1123, #4654, #6557, #3221, #1728, #1680, #6041, #3918, #188, #8100, #5955, #6649, #3873, #3178, #2474, #8701, #8149, #7450, #8794, #2332, #5161, #1075, #8003, #4470, #7308, #3781, #6607, #236, #5907, #2380, #6236, #2623, #8973, #1302, #6977, #6192, #1217, #2709, #3264 ) ),
 .UNSPECIFIED., .F., .F., .F. ) 
 B_SPLINE_SURFACE_WITH_KNOTS ( ( 2, 2 ),
 ( 3, 2, 2, 2, 2, 2, 2, 2, 2, 2, 2, 2, 2, 2, 2, 2, 2, 2, 2, 2, 2, 2, 2, 2, 2, 2, 2, 2, 2, 2, 2, 2, 2, 2, 2, 2, 2, 2, 2, 2, 2, 2, 2, 2, 2, 2, 2, 2, 2, 2, 2, 2, 2, 2, 2, 2, 2, 2, 2, 2, 2, 2, 2, 2, 2, 2, 2, 2, 2, 2, 2, 2, 3 ),
 ( 0.000000000000000000, 1.000000000000000000 ),
 ( 0.000000000000000000, 0.01388888888888888812, 0.02777777777777777624, 0.04166666666666666435, 0.05555555555555555247, 0.06944444444444444753, 0.08333333333333332871, 0.09722222222222222376, 0.1111111111111111049, 0.1250000000000000000, 0.1388888888888888951, 0.1527777777777777901, 0.1666666666666666574, 0.1805555555555555525, 0.1944444444444444475, 0.2083333333333333426, 0.2222222222222222099, 0.2361111111111111049, 0.2500000000000000000, 0.2638888888888888951, 0.2777777777777777901, 0.2916666666666666852, 0.3055555555555555802, 0.3194444444444444198, 0.3333333333333333148, 0.3472222222222222099, 0.3611111111111111049, 0.3750000000000000000, 0.3888888888888888951, 0.4027777777777777901, 0.4166666666666666852, 0.4305555555555555802, 0.4444444444444444198, 0.4583333333333333148, 0.4722222222222222099, 0.4861111111111111049, 0.5000000000000000000, 0.5138888888888888395, 0.5277777777777777901, 0.5416666666666666297, 0.5555555555555555802, 0.5694444444444444198, 0.5833333333333333703, 0.5972222222222222099, 0.6111111111111111605, 0.6250000000000000000, 0.6388888888888888395, 0.6527777777777777901, 0.6666666666666666297, 0.6805555555555555802, 0.6944444444444444198, 0.7083333333333333703, 0.7222222222222222099, 0.7361111111111111605, 0.7500000000000000000, 0.7638888888888888395, 0.7777777777777777901, 0.7916666666666666297, 0.8055555555555555802, 0.8194444444444444198, 0.8333333333333333703, 0.8472222222222222099, 0.8611111111111111605, 0.8750000000000000000, 0.8888888888888888395, 0.9027777777777777901, 0.9166666666666666297, 0.9305555555555555802, 0.9444444444444444198, 0.9583333333333333703, 0.9722222222222222099, 0.9861111111111111605, 1.000000000000000000 ),
 .UNSPECIFIED. ) 
 GEOMETRIC_REPRESENTATION_ITEM ( )  RATIONAL_B_SPLINE_SURFACE ( (
 ( 1.000000000000000000, 0.8660254037844387076, 1.000000000000000000, 0.8660254037844387076, 1.000000000000000000, 0.8660254037844387076, 1.000000000000000000, 0.8660254037844387076, 1.000000000000000000, 0.8660254037844387076, 1.000000000000000000, 0.8660254037844387076, 1.000000000000000000, 0.8660254037844387076, 1.000000000000000000, 0.8660254037844387076, 1.000000000000000000, 0.8660254037844387076, 1.000000000000000000, 0.8660254037844387076, 1.000000000000000000, 0.8660254037844387076, 1.000000000000000000, 0.8660254037844387076, 1.000000000000000000, 0.8660254037844387076, 1.000000000000000000, 0.8660254037844387076, 1.000000000000000000, 0.8660254037844387076, 1.000000000000000000, 0.8660254037844387076, 1.000000000000000000, 0.8660254037844387076, 1.000000000000000000, 0.8660254037844387076, 1.000000000000000000, 0.8660254037844387076, 1.000000000000000000, 0.8660254037844387076, 1.000000000000000000, 0.8660254037844387076, 1.000000000000000000, 0.8660254037844387076, 1.000000000000000000, 0.8660254037844387076, 1.000000000000000000, 0.8660254037844387076, 1.000000000000000000, 0.8660254037844387076, 1.000000000000000000, 0.8660254037844387076, 1.000000000000000000, 0.8660254037844387076, 1.000000000000000000, 0.8660254037844387076, 1.000000000000000000, 0.8660254037844387076, 1.000000000000000000, 0.8660254037844387076, 1.000000000000000000, 0.8660254037844387076, 1.000000000000000000, 0.8660254037844387076, 1.000000000000000000, 0.8660254037844387076, 1.000000000000000000, 0.8660254037844387076, 1.000000000000000000, 0.8660254037844387076, 1.000000000000000000, 0.8660254037844387076, 1.000000000000000000, 0.8660254037844387076, 1.000000000000000000, 0.8660254037844387076, 1.000000000000000000, 0.8660254037844387076, 1.000000000000000000, 0.8660254037844387076, 1.000000000000000000, 0.8660254037844387076, 1.000000000000000000, 0.8660254037844387076, 1.000000000000000000, 0.8660254037844387076, 1.000000000000000000, 0.8660254037844387076, 1.000000000000000000, 0.8660254037844387076, 1.000000000000000000, 0.8660254037844387076, 1.000000000000000000, 0.8660254037844387076, 1.000000000000000000, 0.8660254037844387076, 1.000000000000000000, 0.8660254037844387076, 1.000000000000000000, 0.8660254037844387076, 1.000000000000000000, 0.8660254037844387076, 1.000000000000000000, 0.8660254037844387076, 1.000000000000000000, 0.8660254037844387076, 1.000000000000000000, 0.8660254037844387076, 1.000000000000000000, 0.8660254037844387076, 1.000000000000000000, 0.8660254037844387076, 1.000000000000000000, 0.8660254037844387076, 1.000000000000000000, 0.8660254037844387076, 1.000000000000000000, 0.8660254037844387076, 1.000000000000000000, 0.8660254037844387076, 1.000000000000000000, 0.8660254037844387076, 1.000000000000000000, 0.8660254037844387076, 1.000000000000000000, 0.8660254037844387076, 1.000000000000000000, 0.8660254037844387076, 1.000000000000000000, 0.8660254037844387076, 1.000000000000000000, 0.8660254037844387076, 1.000000000000000000, 0.8660254037844387076, 1.000000000000000000, 0.8660254037844387076, 1.000000000000000000, 0.8660254037844387076, 1.000000000000000000, 0.8660254037844387076, 1.000000000000000000, 0.8660254037844387076, 1.000000000000000000, 0.8660254037844387076, 1.000000000000000000),
 ( 1.000000000000000000, 0.8660254037844387076, 1.000000000000000000, 0.8660254037844387076, 1.000000000000000000, 0.8660254037844387076, 1.000000000000000000, 0.8660254037844387076, 1.000000000000000000, 0.8660254037844387076, 1.000000000000000000, 0.8660254037844387076, 1.000000000000000000, 0.8660254037844387076, 1.000000000000000000, 0.8660254037844387076, 1.000000000000000000, 0.8660254037844387076, 1.000000000000000000, 0.8660254037844387076, 1.000000000000000000, 0.8660254037844387076, 1.000000000000000000, 0.8660254037844387076, 1.000000000000000000, 0.8660254037844387076, 1.000000000000000000, 0.8660254037844387076, 1.000000000000000000, 0.8660254037844387076, 1.000000000000000000, 0.8660254037844387076, 1.000000000000000000, 0.8660254037844387076, 1.000000000000000000, 0.8660254037844387076, 1.000000000000000000, 0.8660254037844387076, 1.000000000000000000, 0.8660254037844387076, 1.000000000000000000, 0.8660254037844387076, 1.000000000000000000, 0.8660254037844387076, 1.000000000000000000, 0.8660254037844387076, 1.000000000000000000, 0.8660254037844387076, 1.000000000000000000, 0.8660254037844387076, 1.000000000000000000, 0.8660254037844387076, 1.000000000000000000, 0.8660254037844387076, 1.000000000000000000, 0.8660254037844387076, 1.000000000000000000, 0.8660254037844387076, 1.000000000000000000, 0.8660254037844387076, 1.000000000000000000, 0.8660254037844387076, 1.000000000000000000, 0.8660254037844387076, 1.000000000000000000, 0.8660254037844387076, 1.000000000000000000, 0.8660254037844387076, 1.000000000000000000, 0.8660254037844387076, 1.000000000000000000, 0.8660254037844387076, 1.000000000000000000, 0.8660254037844387076, 1.000000000000000000, 0.8660254037844387076, 1.000000000000000000, 0.8660254037844387076, 1.000000000000000000, 0.8660254037844387076, 1.000000000000000000, 0.8660254037844387076, 1.000000000000000000, 0.8660254037844387076, 1.000000000000000000, 0.8660254037844387076, 1.000000000000000000, 0.8660254037844387076, 1.000000000000000000, 0.8660254037844387076, 1.000000000000000000, 0.8660254037844387076, 1.000000000000000000, 0.8660254037844387076, 1.000000000000000000, 0.8660254037844387076, 1.000000000000000000, 0.8660254037844387076, 1.000000000000000000, 0.8660254037844387076, 1.000000000000000000, 0.8660254037844387076, 1.000000000000000000, 0.8660254037844387076, 1.000000000000000000, 0.8660254037844387076, 1.000000000000000000, 0.8660254037844387076, 1.000000000000000000, 0.8660254037844387076, 1.000000000000000000, 0.8660254037844387076, 1.000000000000000000, 0.8660254037844387076, 1.000000000000000000, 0.8660254037844387076, 1.000000000000000000, 0.8660254037844387076, 1.000000000000000000, 0.8660254037844387076, 1.000000000000000000, 0.8660254037844387076, 1.000000000000000000, 0.8660254037844387076, 1.000000000000000000, 0.8660254037844387076, 1.000000000000000000, 0.8660254037844387076, 1.000000000000000000, 0.8660254037844387076, 1.000000000000000000, 0.8660254037844387076, 1.000000000000000000, 0.8660254037844387076, 1.000000000000000000, 0.8660254037844387076, 1.000000000000000000, 0.8660254037844387076, 1.000000000000000000, 0.8660254037844387076, 1.000000000000000000, 0.8660254037844387076, 1.000000000000000000, 0.8660254037844387076, 1.000000000000000000) ) ) 
 REPRESENTATION_ITEM ( '' )  SURFACE ( )  );
#8142=EDGE_CURVE ( 'NONE', #627, #7705, #2610, .T. ) ;
#8144=CARTESIAN_POINT ( 'NONE',  ( 2.033577675846918216E-14, -27.31250000000000000, 5.250000000000000888 ) ) ;
#8149=CARTESIAN_POINT ( 'NONE',  ( 2.625000000000000444, -27.45833333333333215, -4.546633369868303021 ) ) ;
#8153=CARTESIAN_POINT ( 'NONE',  ( -5.114683531250000748, -27.02604166700806587, 2.952963913586931888 ) ) ;
#8154=EDGE_LOOP ( 'NONE', ( #495, #5057, #8082, #6144 ) ) ;
#8156=CARTESIAN_POINT ( 'NONE',  ( -5.114683531250000748, -29.50520833367472662, -2.952963913586935440 ) ) ;
#8158=CARTESIAN_POINT ( 'NONE',  ( 9.180150650966086169E-15, -28.59375000068279959, 5.250000000000000000 ) ) ;
#8160=CARTESIAN_POINT ( 'NONE',  ( 2.557341765625000818, -28.13020833367473017, -4.429445870380400052 ) ) ;
#8162=CARTESIAN_POINT ( 'NONE',  ( 2.625000000000000444, -29.20833333333333215, -4.546633369868303021 ) ) ;
#8163=FACE_OUTER_BOUND ( 'NONE', #7328, .T. ) ;
#8164=AXIS2_PLACEMENT_3D ( 'NONE', #7524, #7479, #1862 ) ;
#8169=CARTESIAN_POINT ( 'NONE',  ( 0.000000000000000000, -30.00000000000000000, 0.000000000000000000 ) ) ;
#8175=CARTESIAN_POINT ( 'NONE',  ( 0.000000000000000000, -30.00000000000000000, 0.000000000000000000 ) ) ;
#8176=CARTESIAN_POINT ( 'NONE',  ( 2.624999999999996891, -27.57291666734946389, 4.546633369868304797 ) ) ;
#8178=VERTEX_POINT ( 'NONE', #3703 ) ;
#8182=CARTESIAN_POINT ( 'NONE',  ( -1.406733260263387963, -28.92633545031537068, -5.250000000000001776 ) ) ;
#8187=CARTESIAN_POINT ( 'NONE',  ( 2.624999999999996891, -27.79166666666666430, 4.546633369868304797 ) ) ;
#8195=CARTESIAN_POINT ( 'NONE',  ( 2.625000000000000444, -28.45833333333333215, -4.546633369868303021 ) ) ;
#8202=CARTESIAN_POINT ( 'NONE',  ( -2.557341765625002594, -28.94270833367473017, 4.429445870380399164 ) ) ;
#8204=CARTESIAN_POINT ( 'NONE',  ( -5.250000000000000888, -28.10416666666666785, 3.031088913245533423 ) ) ;
#8205=CARTESIAN_POINT ( 'NONE',  ( -5.114683531250000748, -28.52604166700806587, 2.952963913586931888 ) ) ;
#8206=CARTESIAN_POINT ( 'NONE',  ( -1.975475456537005874E-15, -29.31250000000000000, 5.249999999999999112 ) ) ;
#8207=CARTESIAN_POINT ( 'NONE',  ( -5.249999999999999112, -27.92708333401612819, -3.031088913245536975 ) ) ;
#8208=CARTESIAN_POINT ( 'NONE',  ( 5.114683531250000748, -27.35937500034139802, 0.000000000000000000 ) ) ;
#8211=CARTESIAN_POINT ( 'NONE',  ( 5.204748896376250699E-16, -30.00000000000000000, -4.250000000000000000 ) ) ;
#8220=VERTEX_POINT ( 'NONE', #2450 ) ;
#8222=CARTESIAN_POINT ( 'NONE',  ( 5.250000000000000000, -28.53125000068279604, 0.000000000000000000 ) ) ;
#8225=CIRCLE ( 'NONE', #5836, 5.750000000000000000 ) ;
#8232=DIRECTION ( 'NONE',  ( 0.000000000000000000, 1.000000000000000000, 0.000000000000000000 ) ) ;
#8234=CARTESIAN_POINT ( 'NONE',  ( 5.114683531249999859, -29.33854166700805877, -2.952963913586932776 ) ) ;
#8236=LINE ( 'NONE', #1211, #3627 ) ;
#8239=CARTESIAN_POINT ( 'NONE',  ( 0.000000000000000000, -30.00000000000000000, 4.250000000000000000 ) ) ;
#8243=CARTESIAN_POINT ( 'NONE',  ( -1.975475456537005874E-15, -29.06249999999999645, 5.250000000000000000 ) ) ;
#8246=EDGE_CURVE ( 'NONE', #4614, #6499, #4497, .T. ) ;
#8247=ORIENTED_EDGE ( 'NONE', *, *, #8371, .T. ) ;
#8251=CARTESIAN_POINT ( 'NONE',  ( 2.557341765624996821, -29.65104166700806232, 4.429445870380401828 ) ) ;
#8253=CARTESIAN_POINT ( 'NONE',  ( 0.000000000000000000, -30.00000000000000000, 0.000000000000000000 ) ) ;
#8254=CARTESIAN_POINT ( 'NONE',  ( -5.114683531250000748, -27.02604166700806587, 2.952963913586931888 ) ) ;
#8257=CARTESIAN_POINT ( 'NONE',  ( -1.084901341431563923E-15, -27.67187500034140157, 5.905927827173866440 ) ) ;
#8258=FACE_OUTER_BOUND ( 'NONE', #2406, .T. ) ;
#8259=CARTESIAN_POINT ( 'NONE',  ( 3.616337804771879580E-16, -29.35937500034139802, -5.905927827173866440 ) ) ;
#8268=CARTESIAN_POINT ( 'NONE',  ( -5.250000000000000000, -27.40625000068279604, -6.429395695523604153E-16 ) ) ;
#8277=CARTESIAN_POINT ( 'NONE',  ( 3.616337804771879580E-16, -29.79687500034140157, -5.905927827173866440 ) ) ;
#8278=CARTESIAN_POINT ( 'NONE',  ( 0.000000000000000000, -9.999999999999998224, 0.000000000000000000 ) ) ;
#8283=EDGE_CURVE ( 'NONE', #2547, #3872, #441, .T. ) ;
#8286=DIRECTION ( 'NONE',  ( 0.000000000000000000, 1.000000000000000000, 0.000000000000000000 ) ) ;
#8288=ADVANCED_FACE ( 'NONE', ( #1188 ), #5316, .T. ) ;
#8290=ORIENTED_EDGE ( 'NONE', *, *, #7525, .F. ) ;
#8294=CARTESIAN_POINT ( 'NONE',  ( 5.114683531250000748, -29.60937500034139802, 0.000000000000000000 ) ) ;
#8296=LINE ( 'NONE', #9028, #6881 ) ;
#8297=CARTESIAN_POINT ( 'NONE',  ( 3.616337804771879580E-16, -27.60937500034139802, -5.905927827173866440 ) ) ;
#8302=CARTESIAN_POINT ( 'NONE',  ( 2.557341765625000818, -28.63020833367473017, -4.429445870380400052 ) ) ;
#8303=( BOUNDED_CURVE ( )  B_SPLINE_CURVE ( 2, ( #4070, #7649, #6908, #6204, #9035, #5409, #8350, #434, #3282 ),
 .UNSPECIFIED., .F., .F. ) 
 B_SPLINE_CURVE_WITH_KNOTS ( ( 3, 2, 2, 2, 3 ),
 ( 0.5208333333333332593, 0.5277777777777777901, 0.5416666666666666297, 0.5555555555555555802, 0.5625000000000000000 ),
 .UNSPECIFIED. ) 
 CURVE ( )  GEOMETRIC_REPRESENTATION_ITEM ( )  RATIONAL_B_SPLINE_CURVE ( ( 0.9330127018922192983, 0.9330127018922187432, 1.000000000000000000, 0.8660254037844387076, 1.000000000000000000, 0.8660254037844387076, 1.000000000000000000, 0.9330127018922194093, 0.9330127018922194093 ) ) 
 REPRESENTATION_ITEM ( '' )  );
#8304=CARTESIAN_POINT ( 'NONE',  ( 0.000000000000000000, -9.000000000000001776, 0.000000000000000000 ) ) ;
#8306=DIRECTION ( 'NONE',  ( 0.000000000000000000, 1.000000000000000000, 0.000000000000000000 ) ) ;
#8311=ORIENTED_EDGE ( 'NONE', *, *, #4971, .T. ) ;
#8312=AXIS2_PLACEMENT_3D ( 'NONE', #2515, #926, #4518 ) ;
#8313=CARTESIAN_POINT ( 'NONE',  ( 1.406733260263394625, -29.22991455036742536, -5.250000000000000000 ) ) ;
#8314=CARTESIAN_POINT ( 'NONE',  ( 2.624999999999996891, -28.07291666734946389, 4.546633369868304797 ) ) ;
#8324=CARTESIAN_POINT ( 'NONE',  ( -1.975475456537005874E-15, -28.09375000068279604, 5.250000000000000000 ) ) ;
#8325=CARTESIAN_POINT ( 'NONE',  ( -5.114683531250000748, -29.73437500034139802, -6.263680815196995234E-16 ) ) ;
#8326=DIRECTION ( 'NONE',  ( 0.000000000000000000, 0.000000000000000000, 1.000000000000000000 ) ) ;
#8333=EDGE_CURVE ( 'NONE', #7933, #3248, #2346, .T. ) ;
#8336=VECTOR ( 'NONE', #6894, 1000.000000000000114 ) ;
#8337=CARTESIAN_POINT ( 'NONE',  ( 0.000000000000000000, -30.00000000000000000, 0.000000000000000000 ) ) ;
#8339=ORIENTED_EDGE ( 'NONE', *, *, #4027, .T. ) ;
#8342=AXIS2_PLACEMENT_3D ( 'NONE', #2010, #3363, #6847 ) ;
#8344=CARTESIAN_POINT ( 'NONE',  ( 2.557341765625000818, -28.06770833367473017, -4.429445870380400052 ) ) ;
#8347=CARTESIAN_POINT ( 'NONE',  ( 5.114683531249999859, -27.90104166700806587, -2.952963913586932776 ) ) ;
#8349=CARTESIAN_POINT ( 'NONE',  ( -5.114683531250000748, -28.79687500034139802, -6.263680815196995234E-16 ) ) ;
#8350=CARTESIAN_POINT ( 'NONE',  ( -2.625000000000002220, -28.33333333333333215, 4.546633369868302132 ) ) ;
#8351=CARTESIAN_POINT ( 'NONE',  ( -1.084901341431563923E-15, -29.23437500034139802, 5.905927827173866440 ) ) ;
#8355=CARTESIAN_POINT ( 'NONE',  ( 5.249999999999999112, -29.51041666734945679, -3.031088913245534755 ) ) ;
#8361=CARTESIAN_POINT ( 'NONE',  ( -2.625000000000002220, -27.11458333401612819, 4.546633369868302132 ) ) ;
#8363=( BOUNDED_CURVE ( )  B_SPLINE_CURVE ( 2, ( #2640, #6116, #5511, #4720, #3335, #6865, #8944, #392, #4630 ),
 .UNSPECIFIED., .F., .T. ) 
 B_SPLINE_CURVE_WITH_KNOTS ( ( 3, 2, 2, 2, 3 ),
 ( 0.1875000000000000000, 0.1944444444444444475, 0.2083333333333333426, 0.2222222222222222099, 0.2291666666666666574 ),
 .UNSPECIFIED. ) 
 CURVE ( )  GEOMETRIC_REPRESENTATION_ITEM ( )  RATIONAL_B_SPLINE_CURVE ( ( 0.9330127018922194093, 0.9330127018922194093, 1.000000000000000000, 0.8660254037844387076, 1.000000000000000000, 0.8660254037844387076, 1.000000000000000000, 0.9330127018922194093, 0.9330127018922194093 ) ) 
 REPRESENTATION_ITEM ( '' )  );
#8369=CARTESIAN_POINT ( 'NONE',  ( 9.180150650966086169E-15, -28.59375000068279959, 5.249999999999999112 ) ) ;
#8371=EDGE_CURVE ( 'NONE', #7471, #1378, #4721, .T. ) ;
#8372=CARTESIAN_POINT ( 'NONE',  ( 5.250000000000000000, -28.03125000068279604, 0.000000000000000000 ) ) ;
#8374=CARTESIAN_POINT ( 'NONE',  ( -1.084901341431563923E-15, -28.17187500034139447, 5.905927827173866440 ) ) ;
#8380=VECTOR ( 'NONE', #4338, 1000.000000000000000 ) ;
#8387=CARTESIAN_POINT ( 'NONE',  ( 2.557341765624996821, -27.65104166700806587, 4.429445870380401828 ) ) ;
#8389=CARTESIAN_POINT ( 'NONE',  ( 5.114683531249998971, -26.94270833367472662, 2.952963913586936329 ) ) ;
#8391=EDGE_CURVE ( 'NONE', #2870, #7180, #9056, .T. ) ;
#8392=CARTESIAN_POINT ( 'NONE',  ( 5.114683531250000748, -29.15104166700806232, -2.952963913586932776 ) ) ;
#8395=CARTESIAN_POINT ( 'NONE',  ( 3.616337804771879580E-16, -29.10937500034139447, -5.905927827173866440 ) ) ;
#8402=EDGE_CURVE ( 'NONE', #977, #8760, #5031, .T. ) ;
#8405=CARTESIAN_POINT ( 'NONE',  ( -5.114683531249999859, -29.50520833367473017, -2.952963913586935440 ) ) ;
#8407=ORIENTED_EDGE ( 'NONE', *, *, #6679, .F. ) ;
#8415=CARTESIAN_POINT ( 'NONE',  ( -2.557341765624999042, -28.02604166700806587, -4.429445870380400052 ) ) ;
#8419=DIRECTION ( 'NONE',  ( 0.000000000000000000, 1.000000000000000000, 0.000000000000000000 ) ) ;
#8428=CARTESIAN_POINT ( 'NONE',  ( -5.114683531250001636, -27.21354166700806587, 2.952963913586931444 ) ) ;
#8430=CARTESIAN_POINT ( 'NONE',  ( 2.557341765625000818, -27.88020833367473017, -4.429445870380400052 ) ) ;
#8432=( BOUNDED_CURVE ( )  B_SPLINE_CURVE ( 2, ( #5124, #2957, #2344, #6521, #2204, #1552, #6472, #3695, #4487 ),
 .UNSPECIFIED., .F., .T. ) 
 B_SPLINE_CURVE_WITH_KNOTS ( ( 3, 2, 2, 2, 3 ),
 ( 0.6458333333333333703, 0.6527777777777777901, 0.6666666666666666297, 0.6805555555555555802, 0.6875000000000000000 ),
 .UNSPECIFIED. ) 
 CURVE ( )  GEOMETRIC_REPRESENTATION_ITEM ( )  RATIONAL_B_SPLINE_CURVE ( ( 0.9330127018922192983, 0.9330127018922198534, 1.000000000000000000, 0.8660254037844387076, 1.000000000000000000, 0.8660254037844387076, 1.000000000000000000, 0.9330127018922194093, 0.9330127018922194093 ) ) 
 REPRESENTATION_ITEM ( '' )  );
#8433=CARTESIAN_POINT ( 'NONE',  ( 5.114683531249998971, -29.69270833367473017, 2.952963913586936329 ) ) ;
#8435=CARTESIAN_POINT ( 'NONE',  ( -1.084901341431563923E-15, -28.98437500034139447, 5.905927827173866440 ) ) ;
#8436=CARTESIAN_POINT ( 'NONE',  ( -1.406733260263394847, -29.67633545031537423, -5.250000000000000000 ) ) ;
#8438=CARTESIAN_POINT ( 'NONE',  ( 0.000000000000000000, -30.00000000000000000, 0.000000000000000000 ) ) ;
#8446=CARTESIAN_POINT ( 'NONE',  ( 2.624999999999996891, -27.07291666734946389, 4.546633369868304797 ) ) ;
#8454=EDGE_CURVE ( 'NONE', #5103, #3312, #5442, .T. ) ;
#8460=CARTESIAN_POINT ( 'NONE',  ( 5.114683531249999859, -28.08854166700806232, -2.952963913586932776 ) ) ;
#8462=CARTESIAN_POINT ( 'NONE',  ( 5.249999999999999112, -29.01041666734946389, -3.031088913245534755 ) ) ;
#8469=PLANE ( 'NONE',  #3738 ) ;
#8470=CARTESIAN_POINT ( 'NONE',  ( 2.033577675846918216E-14, -26.84375000068279959, 5.250000000000000888 ) ) ;
#8476=CARTESIAN_POINT ( 'NONE',  ( -2.557341765624999042, -27.52604166700806587, -4.429445870380400052 ) ) ;
#8479=CARTESIAN_POINT ( 'NONE',  ( 2.624999999999996891, -29.79166666666666430, 4.546633369868304797 ) ) ;
#8481=CARTESIAN_POINT ( 'NONE',  ( 5.114683531250000748, -29.67187500034139802, 0.000000000000000000 ) ) ;
#8482=MECHANICAL_DESIGN_GEOMETRIC_PRESENTATION_REPRESENTATION('',(#3292),#4452);
#8484=CARTESIAN_POINT ( 'NONE',  ( -1.084901341431563923E-15, -27.23437500034139802, 5.905927827173866440 ) ) ;
#8485=CARTESIAN_POINT ( 'NONE',  ( -1.406733260263390628, -28.35491455036742181, 5.250000000000001776 ) ) ;
#8489=CARTESIAN_POINT ( 'NONE',  ( -1.975475456537005874E-15, -29.81249999999999645, 5.249999999999999112 ) ) ;
#8491=( BOUNDED_CURVE ( )  B_SPLINE_CURVE ( 2, ( #2097, #6361, #1573, #4236, #2227, #3582, #7066, #2849, #8470 ),
 .UNSPECIFIED., .F., .T. ) 
 B_SPLINE_CURVE_WITH_KNOTS ( ( 3, 2, 2, 2, 3 ),
 ( 0.9375000000000000000, 0.9444444444444444198, 0.9583333333333333703, 0.9722222222222222099, 0.9791666666666667407 ),
 .UNSPECIFIED. ) 
 CURVE ( )  GEOMETRIC_REPRESENTATION_ITEM ( )  RATIONAL_B_SPLINE_CURVE ( ( 0.9330127018922194093, 0.9330127018922194093, 1.000000000000000000, 0.8660254037844387076, 1.000000000000000000, 0.8660254037844387076, 1.000000000000000000, 0.9330127018922187432, 0.9330127018922192983 ) ) 
 REPRESENTATION_ITEM ( '' )  );
#8492=VERTEX_POINT ( 'NONE', #4206 ) ;
#8495=CARTESIAN_POINT ( 'NONE',  ( -5.114683531249999859, -29.75520833367473017, -2.952963913586935440 ) ) ;
#8505=CARTESIAN_POINT ( 'NONE',  ( -5.114683531249999859, -29.25520833367473017, -2.952963913586935440 ) ) ;
#8512=CIRCLE ( 'NONE', #336, 4.250000000000000000 ) ;
#8519=CARTESIAN_POINT ( 'NONE',  ( 2.557341765625000818, -28.31770833367473017, -4.429445870380400052 ) ) ;
#8521=CARTESIAN_POINT ( 'NONE',  ( -2.624999999999998668, -29.66666666666666430, -4.546633369868303021 ) ) ;
#8523=EDGE_CURVE ( 'NONE', #6529, #8492, #6077, .T. ) ;
#8524=CARTESIAN_POINT ( 'NONE',  ( -1.084901341431563726E-15, -29.23437500034139802, 5.905927827173866440 ) ) ;
#8525=CARTESIAN_POINT ( 'NONE',  ( -2.557341765624999042, -28.33854166700806587, -4.429445870380400052 ) ) ;
#8534=CARTESIAN_POINT ( 'NONE',  ( 5.114683531250000748, -29.85937500034139802, 0.000000000000000000 ) ) ;
#8536=EDGE_CURVE ( 'NONE', #3111, #813, #6384, .T. ) ;
#8543=CARTESIAN_POINT ( 'NONE',  ( 6.429395695523604153E-16, 75.00000000000000000, -5.250000000000000000 ) ) ;
#8544=CARTESIAN_POINT ( 'NONE',  ( 6.972266317189433020E-16, -27.93749999999999289, -5.249999999999999112 ) ) ;
#8545=CARTESIAN_POINT ( 'NONE',  ( -5.114683531249999859, -28.50520833367473017, -2.952963913586935440 ) ) ;
#8547=CARTESIAN_POINT ( 'NONE',  ( -5.250000000000000888, -28.88541666734946389, 3.031088913245533423 ) ) ;
#8549=CARTESIAN_POINT ( 'NONE',  ( -2.624999999999998668, -28.19791666734946389, -4.546633369868303021 ) ) ;
#8552=( NAMED_UNIT ( * ) PLANE_ANGLE_UNIT ( ) SI_UNIT ( $, .RADIAN. ) );
#8553=CARTESIAN_POINT ( 'NONE',  ( -2.624999999999998668, -27.69791666734946389, -4.546633369868303021 ) ) ;
#8561=CARTESIAN_POINT ( 'NONE',  ( -2.624999999999998668, -29.41666666666666785, -4.546633369868303021 ) ) ;
#8564=CARTESIAN_POINT ( 'NONE',  ( -2.557341765625002594, -27.50520833367473017, 4.429445870380399164 ) ) ;
#8566=CARTESIAN_POINT ( 'NONE',  ( -5.114683531250000748, -27.54687500034139802, -6.263680815196995234E-16 ) ) ;
#8567=CYLINDRICAL_SURFACE ( 'NONE', #5828, 5.250000000000000000 ) ;
#8571=CARTESIAN_POINT ( 'NONE',  ( -2.557341765625002594, -29.75520833367473017, 4.429445870380399164 ) ) ;
#8572=MECHANICAL_DESIGN_GEOMETRIC_PRESENTATION_REPRESENTATION('',(#5742),#3981);
#8576=CARTESIAN_POINT ( 'NONE',  ( 5.249999999999999112, -27.01041666734946389, -3.031088913245534755 ) ) ;
#8577=CARTESIAN_POINT ( 'NONE',  ( 5.114683531250000748, -28.10937500034139447, 0.000000000000000000 ) ) ;
#8578=ORIENTED_EDGE ( 'NONE', *, *, #3331, .T. ) ;
#8581=CARTESIAN_POINT ( 'NONE',  ( 5.249999999999997335, -26.80208333401613174, 3.031088913245538308 ) ) ;
#8587=CARTESIAN_POINT ( 'NONE',  ( -2.557341765625002594, -27.69270833367473017, 4.429445870380399164 ) ) ;
#8595=CARTESIAN_POINT ( 'NONE',  ( 1.406733260263394625, -27.19866454968463287, -5.250000000000000000 ) ) ;
#8597=DIRECTION ( 'NONE',  ( 0.000000000000000000, 1.000000000000000000, 0.000000000000000000 ) ) ;
#8605=CARTESIAN_POINT ( 'NONE',  ( 5.249999999999999112, -28.52083333333333215, 3.031088913245538308 ) ) ;
#8606=ADVANCED_FACE ( 'NONE', ( #6656 ), #4339, .T. ) ;
#8608=CARTESIAN_POINT ( 'NONE',  ( -5.114683531250000748, -27.31770833367473017, -2.952963913586935440 ) ) ;
#8610=CARTESIAN_POINT ( 'NONE',  ( 3.616337804771879580E-16, -27.85937500034139802, -5.905927827173866440 ) ) ;
#8612=DIRECTION ( 'NONE',  ( 0.000000000000000000, 1.000000000000000000, 0.000000000000000000 ) ) ;
#8616=CARTESIAN_POINT ( 'NONE',  ( -2.557341765625002594, -29.50520833367473017, 4.429445870380399164 ) ) ;
#8620=CARTESIAN_POINT ( 'NONE',  ( 2.033577675846918216E-14, -27.09375000068279604, 5.250000000000000888 ) ) ;
#8621=CIRCLE ( 'NONE', #4616, 4.250000000000000000 ) ;
#8622=CARTESIAN_POINT ( 'NONE',  ( -5.114683531249999859, -28.00520833367473017, -2.952963913586935440 ) ) ;
#8628=CARTESIAN_POINT ( 'NONE',  ( -1.975475456537005874E-15, -27.56249999999999289, 5.250000000000000000 ) ) ;
#8630=ORIENTED_EDGE ( 'NONE', *, *, #3665, .T. ) ;
#8632=CARTESIAN_POINT ( 'NONE',  ( -1.406733260263393293, -29.92633545031536713, -5.250000000000000000 ) ) ;
#8633=CARTESIAN_POINT ( 'NONE',  ( -5.250000000000000000, -28.92708333401613174, -3.031088913245536531 ) ) ;
#8634=CARTESIAN_POINT ( 'NONE',  ( 5.249999999999997335, -27.80208333401612819, 3.031088913245538308 ) ) ;
#8635=CARTESIAN_POINT ( 'NONE',  ( 2.557341765625000818, -27.31770833367473017, -4.429445870380400052 ) ) ;
#8638=DIRECTION ( 'NONE',  ( 1.000000000000000000, 0.000000000000000000, 0.000000000000000000 ) ) ;
#8642=DIRECTION ( 'NONE',  ( 0.000000000000000000, 0.000000000000000000, 1.000000000000000000 ) ) ;
#8643=( BOUNDED_CURVE ( )  B_SPLINE_CURVE ( 2, ( #4203, #8436, #620, #7741, #1364, #4560, #5293, #273, #5341 ),
 .UNSPECIFIED., .F., .F. ) 
 B_SPLINE_CURVE_WITH_KNOTS ( ( 3, 2, 2, 2, 3 ),
 ( 0.1041666666666666713, 0.1111111111111111049, 0.1250000000000000000, 0.1388888888888888951, 0.1458333333333333426 ),
 .UNSPECIFIED. ) 
 CURVE ( )  GEOMETRIC_REPRESENTATION_ITEM ( )  RATIONAL_B_SPLINE_CURVE ( ( 0.9330127018922194093, 0.9330127018922194093, 1.000000000000000000, 0.8660254037844387076, 1.000000000000000000, 0.8660254037844387076, 1.000000000000000000, 0.9330127018922194093, 0.9330127018922194093 ) ) 
 REPRESENTATION_ITEM ( '' )  );
#8645=VERTEX_POINT ( 'NONE', #5771 ) ;
#8649=ORIENTED_EDGE ( 'NONE', *, *, #8402, .F. ) ;
#8652=ORIENTED_EDGE ( 'NONE', *, *, #4138, .T. ) ;
#8653=CARTESIAN_POINT ( 'NONE',  ( -2.625000000000002220, -28.83333333333333215, 4.546633369868302132 ) ) ;
#8654=CARTESIAN_POINT ( 'NONE',  ( 5.250000000000000000, -29.75000000000000000, 0.000000000000000000 ) ) ;
#8655=CARTESIAN_POINT ( 'NONE',  ( -5.114683531250001636, -28.02604166700806587, 2.952963913586931444 ) ) ;
#8658=CARTESIAN_POINT ( 'NONE',  ( -2.557341765624999042, -27.33854166700806587, -4.429445870380400052 ) ) ;
#8663=AXIS2_PLACEMENT_3D ( 'NONE', #1451, #895, #2339 ) ;
#8664=CARTESIAN_POINT ( 'NONE',  ( -2.624999999999998668, -29.69791666734946034, -4.546633369868303021 ) ) ;
#8666=ORIENTED_EDGE ( 'NONE', *, *, #3134, .T. ) ;
#8668=CARTESIAN_POINT ( 'NONE',  ( 1.406733260263394625, -26.97991455036742181, -5.250000000000000000 ) ) ;
#8669=CARTESIAN_POINT ( 'NONE',  ( 5.114683531249999859, -28.58854166700806232, -2.952963913586932776 ) ) ;
#8679=CARTESIAN_POINT ( 'NONE',  ( -2.624999999999998668, -29.44791666734946034, -4.546633369868303021 ) ) ;
#8681=CARTESIAN_POINT ( 'NONE',  ( -5.114683531250000748, -27.46354166700806232, 2.952963913586931888 ) ) ;
#8685=UNCERTAINTY_MEASURE_WITH_UNIT (LENGTH_MEASURE( 1.000000000000000082E-05 ), #1080, 'distance_accuracy_value', 'NONE');
#8698=FACE_OUTER_BOUND ( 'NONE', #339, .T. ) ;
#8701=CARTESIAN_POINT ( 'NONE',  ( 5.250000000000000000, -27.47916666666666430, -3.031088913245534755 ) ) ;
#8702=CARTESIAN_POINT ( 'NONE',  ( -2.557341765625002594, -28.00520833367473017, 4.429445870380399164 ) ) ;
#8703=SHAPE_REPRESENTATION_RELATIONSHIP ( 'NONE' , 'NONE' ,  #4551, #4641 ) ;
#8714=CARTESIAN_POINT ( 'NONE',  ( -5.114683531250000748, -28.73437500034139802, -6.263680815196995234E-16 ) ) ;
#8719=EDGE_CURVE ( 'NONE', #7275, #803, #3830, .T. ) ;
#8721=EDGE_LOOP ( 'NONE', ( #202, #163, #7368 ) ) ;
#8723=CARTESIAN_POINT ( 'NONE',  ( -5.250000000000000888, -28.88541666734946745, 3.031088913245532979 ) ) ;
#8724=( BOUNDED_CURVE ( )  B_SPLINE_CURVE ( 2, ( #6160, #338, #3192, #700, #1974, #4885, #5631, #4972, #3372, #1361, #4805, #8433, #8481, #9164, #5589, #532, #4112, #617, #7826, #1443, #5675, #5547, #7077, #7689, #9034, #3504, #6369, #9080, #7647, #4844, #2105, #7784, #3458, #8524, #6944, #4929, #6203, #8392, #4288, #9123, #1404, #6990, #2676, #4244, #1274, #3545, #7737, #1313, #661, #9, #5505, #4200, #6289, #2859, #8349, #573, #4154, #3418, #6327, #7036, #2151, #6248, #2721, #2019, #2769, #2059, #2811, #934, #746, #5817, #7309, #8006, #55, #4381, #6608, #189, #1681, #237, #7869, #1585, #7961, #4335, #3044, #7122, #2946, #2382, #6507, #1634, #5862, #94, #7213, #8655, #8702, #2333, #1491, #7168, #3683, #5063, #5211, #3086, #5163, #6415, #3592, #1540, #2903, #3736, #4426, #3783, #143, #4472, #5909, #8750, #7916, #5720, #2995, #8054, #8564, #2287, #2192, #5014, #795, #3639, #6462, #837, #5765, #8608, #2240, #5113, #7259, #887, #6559, #6147, #8928, #4656, #3966, #5348, #6697, #375, #3223, #2523, #3179, #1078, #1879, #2429, #325 ),
 .UNSPECIFIED., .F., .F. ) 
 B_SPLINE_CURVE_WITH_KNOTS ( ( 3, 2, 2, 2, 2, 2, 2, 2, 2, 2, 2, 2, 2, 2, 2, 2, 2, 2, 2, 2, 2, 2, 2, 2, 2, 2, 2, 2, 2, 2, 2, 2, 2, 2, 2, 2, 2, 2, 2, 2, 2, 2, 2, 2, 2, 2, 2, 2, 2, 2, 2, 2, 2, 2, 2, 2, 2, 2, 2, 2, 2, 2, 2, 2, 2, 2, 2, 2, 2, 2, 2, 2, 3 ),
 ( 0.000000000000000000, 0.01388888888888888812, 0.02777777777777777624, 0.04166666666666666435, 0.05555555555555555247, 0.06944444444444444753, 0.08333333333333332871, 0.09722222222222222376, 0.1111111111111111049, 0.1250000000000000000, 0.1388888888888888951, 0.1527777777777777901, 0.1666666666666666574, 0.1805555555555555525, 0.1944444444444444475, 0.2083333333333333426, 0.2222222222222222099, 0.2361111111111111049, 0.2500000000000000000, 0.2638888888888888951, 0.2777777777777777901, 0.2916666666666666852, 0.3055555555555555802, 0.3194444444444444198, 0.3333333333333333148, 0.3472222222222222099, 0.3611111111111111049, 0.3750000000000000000, 0.3888888888888888951, 0.4027777777777777901, 0.4166666666666666852, 0.4305555555555555802, 0.4444444444444444198, 0.4583333333333333148, 0.4722222222222222099, 0.4861111111111111049, 0.5000000000000000000, 0.5138888888888888395, 0.5277777777777777901, 0.5416666666666666297, 0.5555555555555555802, 0.5694444444444444198, 0.5833333333333333703, 0.5972222222222222099, 0.6111111111111111605, 0.6250000000000000000, 0.6388888888888888395, 0.6527777777777777901, 0.6666666666666666297, 0.6805555555555555802, 0.6944444444444444198, 0.7083333333333333703, 0.7222222222222222099, 0.7361111111111111605, 0.7500000000000000000, 0.7638888888888888395, 0.7777777777777777901, 0.7916666666666666297, 0.8055555555555555802, 0.8194444444444444198, 0.8333333333333333703, 0.8472222222222222099, 0.8611111111111111605, 0.8750000000000000000, 0.8888888888888888395, 0.9027777777777777901, 0.9166666666666666297, 0.9305555555555555802, 0.9444444444444444198, 0.9583333333333333703, 0.9722222222222222099, 0.9861111111111111605, 1.000000000000000000 ),
 .UNSPECIFIED. ) 
 CURVE ( )  GEOMETRIC_REPRESENTATION_ITEM ( )  RATIONAL_B_SPLINE_CURVE ( ( 1.000000000000000000, 0.8660254037844387076, 1.000000000000000000, 0.8660254037844387076, 1.000000000000000000, 0.8660254037844387076, 1.000000000000000000, 0.8660254037844387076, 1.000000000000000000, 0.8660254037844387076, 1.000000000000000000, 0.8660254037844387076, 1.000000000000000000, 0.8660254037844387076, 1.000000000000000000, 0.8660254037844387076, 1.000000000000000000, 0.8660254037844387076, 1.000000000000000000, 0.8660254037844387076, 1.000000000000000000, 0.8660254037844387076, 1.000000000000000000, 0.8660254037844387076, 1.000000000000000000, 0.8660254037844387076, 1.000000000000000000, 0.8660254037844387076, 1.000000000000000000, 0.8660254037844387076, 1.000000000000000000, 0.8660254037844387076, 1.000000000000000000, 0.8660254037844387076, 1.000000000000000000, 0.8660254037844387076, 1.000000000000000000, 0.8660254037844387076, 1.000000000000000000, 0.8660254037844387076, 1.000000000000000000, 0.8660254037844387076, 1.000000000000000000, 0.8660254037844387076, 1.000000000000000000, 0.8660254037844387076, 1.000000000000000000, 0.8660254037844387076, 1.000000000000000000, 0.8660254037844387076, 1.000000000000000000, 0.8660254037844387076, 1.000000000000000000, 0.8660254037844387076, 1.000000000000000000, 0.8660254037844387076, 1.000000000000000000, 0.8660254037844387076, 1.000000000000000000, 0.8660254037844387076, 1.000000000000000000, 0.8660254037844387076, 1.000000000000000000, 0.8660254037844387076, 1.000000000000000000, 0.8660254037844387076, 1.000000000000000000, 0.8660254037844387076, 1.000000000000000000, 0.8660254037844387076, 1.000000000000000000, 0.8660254037844387076, 1.000000000000000000, 0.8660254037844387076, 1.000000000000000000, 0.8660254037844387076, 1.000000000000000000, 0.8660254037844387076, 1.000000000000000000, 0.8660254037844387076, 1.000000000000000000, 0.8660254037844387076, 1.000000000000000000, 0.8660254037844387076, 1.000000000000000000, 0.8660254037844387076, 1.000000000000000000, 0.8660254037844387076, 1.000000000000000000, 0.8660254037844387076, 1.000000000000000000, 0.8660254037844387076, 1.000000000000000000, 0.8660254037844387076, 1.000000000000000000, 0.8660254037844387076, 1.000000000000000000, 0.8660254037844387076, 1.000000000000000000, 0.8660254037844387076, 1.000000000000000000, 0.8660254037844387076, 1.000000000000000000, 0.8660254037844387076, 1.000000000000000000, 0.8660254037844387076, 1.000000000000000000, 0.8660254037844387076, 1.000000000000000000, 0.8660254037844387076, 1.000000000000000000, 0.8660254037844387076, 1.000000000000000000, 0.8660254037844387076, 1.000000000000000000, 0.8660254037844387076, 1.000000000000000000, 0.8660254037844387076, 1.000000000000000000, 0.8660254037844387076, 1.000000000000000000, 0.8660254037844387076, 1.000000000000000000, 0.8660254037844387076, 1.000000000000000000, 0.8660254037844387076, 1.000000000000000000, 0.8660254037844387076, 1.000000000000000000, 0.8660254037844387076, 1.000000000000000000, 0.8660254037844387076, 1.000000000000000000, 0.8660254037844387076, 1.000000000000000000, 0.8660254037844387076, 1.000000000000000000, 0.8660254037844387076, 1.000000000000000000, 0.8660254037844387076, 1.000000000000000000, 0.8660254037844387076, 1.000000000000000000, 0.8660254037844387076, 1.000000000000000000 ) ) 
 REPRESENTATION_ITEM ( '' )  );
#8726=CARTESIAN_POINT ( 'NONE',  ( 2.557341765624996821, -26.90104166700806232, 4.429445870380401828 ) ) ;
#8731=CARTESIAN_POINT ( 'NONE',  ( 6.429395695523604153E-16, -9.000000000000001776, -5.250000000000000000 ) ) ;
#8741=CARTESIAN_POINT ( 'NONE',  ( -2.625000000000002220, -27.33333333333333215, 4.546633369868302132 ) ) ;
#8746=CARTESIAN_POINT ( 'NONE',  ( -5.250000000000000888, -28.35416666666666785, 3.031088913245532979 ) ) ;
#8750=CARTESIAN_POINT ( 'NONE',  ( 3.616337804771879580E-16, -27.60937500034139802, -5.905927827173866440 ) ) ;
#8754=CARTESIAN_POINT ( 'NONE',  ( 2.557341765625000818, -29.81770833367473372, -4.429445870380400052 ) ) ;
#8758=CARTESIAN_POINT ( 'NONE',  ( 3.616337804771879580E-16, -29.35937500034139802, -5.905927827173866440 ) ) ;
#8759=DIRECTION ( 'NONE',  ( 0.000000000000000000, 0.000000000000000000, 1.000000000000000000 ) ) ;
#8760=VERTEX_POINT ( 'NONE', #6704 ) ;
#8763=CARTESIAN_POINT ( 'NONE',  ( 2.557341765624996821, -28.15104166700806587, 4.429445870380401828 ) ) ;
#8764=ORIENTED_EDGE ( 'NONE', *, *, #3959, .T. ) ;
#8765=CARTESIAN_POINT ( 'NONE',  ( 0.000000000000000000, -30.00000000000000000, 0.000000000000000000 ) ) ;
#8773=CARTESIAN_POINT ( 'NONE',  ( 3.712013335537174572E-16, -28.96875000068279959, -6.062177826491070398 ) ) ;
#8775=CARTESIAN_POINT ( 'NONE',  ( 5.114683531250000748, -27.10937500034139802, 0.000000000000000000 ) ) ;
#8781=( BOUNDED_CURVE ( )  B_SPLINE_CURVE ( 2, ( #1292, #2653, #4781, #1865, #4689, #6779, #7527, #7623, #1154 ),
 .UNSPECIFIED., .F., .F. ) 
 B_SPLINE_CURVE_WITH_KNOTS ( ( 3, 2, 2, 2, 3 ),
 ( 0.5625000000000000000, 0.5694444444444444198, 0.5833333333333333703, 0.5972222222222222099, 0.6041666666666666297 ),
 .UNSPECIFIED. ) 
 CURVE ( )  GEOMETRIC_REPRESENTATION_ITEM ( )  RATIONAL_B_SPLINE_CURVE ( ( 0.9330127018922194093, 0.9330127018922194093, 1.000000000000000000, 0.8660254037844387076, 1.000000000000000000, 0.8660254037844387076, 1.000000000000000000, 0.9330127018922198534, 0.9330127018922192983 ) ) 
 REPRESENTATION_ITEM ( '' )  );
#8786=DIRECTION ( 'NONE',  ( 0.000000000000000000, 1.000000000000000000, 0.000000000000000000 ) ) ;
#8789=CARTESIAN_POINT ( 'NONE',  ( -5.250000000000000888, -27.35416666666666430, 3.031088913245533423 ) ) ;
#8790=ORIENTED_EDGE ( 'NONE', *, *, #8067, .T. ) ;
#8793=ORIENTED_EDGE ( 'NONE', *, *, #1794, .F. ) ;
#8794=CARTESIAN_POINT ( 'NONE',  ( -2.624999999999998668, -27.41666666666666430, -4.546633369868303021 ) ) ;
#8798=ORIENTED_EDGE ( 'NONE', *, *, #1859, .T. ) ;
#8799=CARTESIAN_POINT ( 'NONE',  ( 2.557341765624996821, -29.40104166700806232, 4.429445870380401828 ) ) ;
#8801=CARTESIAN_POINT ( 'NONE',  ( 1.406733260263394625, -28.47991455036742892, -5.250000000000000000 ) ) ;
#8802=CARTESIAN_POINT ( 'NONE',  ( -2.557341765624999042, -28.58854166700806587, -4.429445870380400052 ) ) ;
#8807=CARTESIAN_POINT ( 'NONE',  ( 5.114683531249999859, -27.58854166700806587, -2.952963913586932776 ) ) ;
#8808=VERTEX_POINT ( 'NONE', #6755 ) ;
#8809=VECTOR ( 'NONE', #8232, 1000.000000000000000 ) ;
#8816=CARTESIAN_POINT ( 'NONE',  ( -2.624999999999998668, -29.91666666666666430, -4.546633369868303021 ) ) ;
#8818=EDGE_CURVE ( 'NONE', #2168, #8837, #8053, .T. ) ;
#8820=AXIS2_PLACEMENT_3D ( 'NONE', #4408, #6488, #1566 ) ;
#8824=DIRECTION ( 'NONE',  ( 1.000000000000000000, 0.000000000000000000, 0.000000000000000000 ) ) ;
#8829=CARTESIAN_POINT ( 'NONE',  ( -5.114683531249999859, -29.75520833367473017, -2.952963913586935440 ) ) ;
#8830=ORIENTED_EDGE ( 'NONE', *, *, #1730, .F. ) ;
#8834=ORIENTED_EDGE ( 'NONE', *, *, #4748, .T. ) ;
#8837=VERTEX_POINT ( 'NONE', #1787 ) ;
#8838=CARTESIAN_POINT ( 'NONE',  ( -5.250000000000000888, -27.85416666666666430, 3.031088913245532979 ) ) ;
#8842=VERTEX_POINT ( 'NONE', #2437 ) ;
#8844=CARTESIAN_POINT ( 'NONE',  ( 2.557341765625000818, -29.06770833367473017, -4.429445870380400052 ) ) ;
#8848=CARTESIAN_POINT ( 'NONE',  ( 5.114683531249998971, -28.19270833367473372, 2.952963913586936329 ) ) ;
#8850=CARTESIAN_POINT ( 'NONE',  ( -2.557341765624999042, -27.77604166700806587, -4.429445870380400052 ) ) ;
#8859=CARTESIAN_POINT ( 'NONE',  ( 5.249999999999999112, -28.05208333401612819, 3.031088913245538308 ) ) ;
#8861=ORIENTED_EDGE ( 'NONE', *, *, #2193, .F. ) ;
#8869=CARTESIAN_POINT ( 'NONE',  ( 2.557341765624996821, -29.40104166700806232, 4.429445870380401828 ) ) ;
#8877=ORIENTED_EDGE ( 'NONE', *, *, #2827, .F. ) ;
#8878=CARTESIAN_POINT ( 'NONE',  ( -2.625000000000002220, -27.83333333333333215, 4.546633369868302132 ) ) ;
#8886=VECTOR ( 'NONE', #1475, 1000.000000000000000 ) ;
#8887=CARTESIAN_POINT ( 'NONE',  ( 2.557341765625000818, -29.31770833367473017, -4.429445870380400052 ) ) ;
#8891=CARTESIAN_POINT ( 'NONE',  ( 2.557341765624996821, -28.71354166700806587, 4.429445870380401828 ) ) ;
#8892=EDGE_CURVE ( 'NONE', #3365, #6742, #2225, .T. ) ;
#8893=CARTESIAN_POINT ( 'NONE',  ( -1.406733260263385521, -27.85491455036742536, 5.250000000000006217 ) ) ;
#8896=ORIENTED_EDGE ( 'NONE', *, *, #3394, .F. ) ;
#8902=ORIENTED_EDGE ( 'NONE', *, *, #79, .F. ) ;
#8905=CARTESIAN_POINT ( 'NONE',  ( -1.113604000661152470E-15, -27.84375000068279604, 6.062177826491070398 ) ) ;
#8914=CARTESIAN_POINT ( 'NONE',  ( -2.624999999999998668, -28.91666666666666785, -4.546633369868303021 ) ) ;
#8917=DIRECTION ( 'NONE',  ( -0.000000000000000000, -1.000000000000000000, -0.000000000000000000 ) ) ;
#8926=CARTESIAN_POINT ( 'NONE',  ( -2.624999999999998668, -27.19791666734946389, -4.546633369868303021 ) ) ;
#8927=DIRECTION ( 'NONE',  ( 0.000000000000000000, 0.000000000000000000, 1.000000000000000000 ) ) ;
#8928=CARTESIAN_POINT ( 'NONE',  ( 5.114683531250000748, -27.17187500034139802, 0.000000000000000000 ) ) ;
#8929=VERTEX_POINT ( 'NONE', #3862 ) ;
#8932=CARTESIAN_POINT ( 'NONE',  ( -5.114683531250000748, -29.48437500034139802, -6.263680815196995234E-16 ) ) ;
#8934=CARTESIAN_POINT ( 'NONE',  ( 2.033577675846918216E-14, -28.06249999999999645, 5.250000000000000888 ) ) ;
#8935=CARTESIAN_POINT ( 'NONE',  ( -5.114683531250000748, -29.29687500034139802, -6.263680815196995234E-16 ) ) ;
#8936=CARTESIAN_POINT ( 'NONE',  ( 5.249999999999999112, -29.22916666666666785, -3.031088913245534755 ) ) ;
#8937=DIRECTION ( 'NONE',  ( 0.000000000000000000, 0.000000000000000000, 1.000000000000000000 ) ) ;
#8938=CARTESIAN_POINT ( 'NONE',  ( 5.249999999999997335, -27.02083333333334281, 3.031088913245538308 ) ) ;
#8939=CARTESIAN_POINT ( 'NONE',  ( 5.114683531250000748, -29.42187500034139802, 0.000000000000000000 ) ) ;
#8940=( BOUNDED_CURVE ( )  B_SPLINE_CURVE ( 2, ( #2815, #3462, #9037, #6372, #4246, #4932, #1977, #8485, #2062 ),
 .UNSPECIFIED., .F., .F. ) 
 B_SPLINE_CURVE_WITH_KNOTS ( ( 3, 2, 2, 2, 3 ),
 ( 0.4375000000000000000, 0.4444444444444444198, 0.4583333333333333148, 0.4722222222222222099, 0.4791666666666666852 ),
 .UNSPECIFIED. ) 
 CURVE ( )  GEOMETRIC_REPRESENTATION_ITEM ( )  RATIONAL_B_SPLINE_CURVE ( ( 0.9330127018922194093, 0.9330127018922194093, 1.000000000000000000, 0.8660254037844387076, 1.000000000000000000, 0.8660254037844387076, 1.000000000000000000, 0.9330127018922190762, 0.9330127018922194093 ) ) 
 REPRESENTATION_ITEM ( '' )  );
#8944=CARTESIAN_POINT ( 'NONE',  ( -2.625000000000002220, -29.11458333401613174, 4.546633369868302132 ) ) ;
#8951=CARTESIAN_POINT ( 'NONE',  ( -5.250000000000000000, -27.65625000068279959, -6.429395695523604153E-16 ) ) ;
#8958=FACE_OUTER_BOUND ( 'NONE', #7818, .T. ) ;
#8961=CARTESIAN_POINT ( 'NONE',  ( 9.180150650966086169E-15, -28.81250000000000000, 5.250000000000000000 ) ) ;
#8965=ORIENTED_EDGE ( 'NONE', *, *, #7129, .F. ) ;
#8969=DIRECTION ( 'NONE',  ( 0.000000000000000000, 1.000000000000000000, 0.000000000000000000 ) ) ;
#8973=CARTESIAN_POINT ( 'NONE',  ( -5.250000000000000000, -27.12500000000000000, -6.429395695523604153E-16 ) ) ;
#8977=ORIENTED_EDGE ( 'NONE', *, *, #513, .T. ) ;
#8980=EDGE_LOOP ( 'NONE', ( #2303, #45, #6892, #8861 ) ) ;
#8981=CARTESIAN_POINT ( 'NONE',  ( -5.114683531250000748, -28.98437500034139802, -6.263680815196995234E-16 ) ) ;
#8983=DIRECTION ( 'NONE',  ( 0.000000000000000000, 1.000000000000000000, 0.000000000000000000 ) ) ;
#8984=CARTESIAN_POINT ( 'NONE',  ( 2.557341765624996821, -27.21354166700806587, 4.429445870380401828 ) ) ;
#8986=CARTESIAN_POINT ( 'NONE',  ( 2.557341765625000818, -27.56770833367473017, -4.429445870380400052 ) ) ;
#8987=DIRECTION ( 'NONE',  ( 0.000000000000000000, 1.000000000000000000, 0.000000000000000000 ) ) ;
#8988=CARTESIAN_POINT ( 'NONE',  ( 5.114683531249998971, -29.19270833367473017, 2.952963913586936329 ) ) ;
#8991=CARTESIAN_POINT ( 'NONE',  ( 0.000000000000000000, -30.00000000000000000, 0.000000000000000000 ) ) ;
#8997=CARTESIAN_POINT ( 'NONE',  ( 6.972266317189433020E-16, -29.21875000068279249, -5.250000000000000000 ) ) ;
#8998=CARTESIAN_POINT ( 'NONE',  ( -5.250000000000000000, -28.67708333401612819, -3.031088913245536531 ) ) ;
#9005=CARTESIAN_POINT ( 'NONE',  ( 5.249999999999999112, -29.76041666734946034, -3.031088913245534755 ) ) ;
#9009=CARTESIAN_POINT ( 'NONE',  ( 2.624999999999996891, -28.07291666734946389, 4.546633369868304797 ) ) ;
#9012=CARTESIAN_POINT ( 'NONE',  ( 0.000000000000000000, -9.000000000000000000, 0.000000000000000000 ) ) ;
#9020=LINE ( 'NONE', #7540, #3614 ) ;
#9021=DIRECTION ( 'NONE',  ( 0.000000000000000000, 1.000000000000000000, 0.000000000000000000 ) ) ;
#9026=CARTESIAN_POINT ( 'NONE',  ( 2.557341765625000818, -27.06770833367473017, -4.429445870380400052 ) ) ;
#9028=CARTESIAN_POINT ( 'NONE',  ( 6.429395695523604153E-16, -30.00000000000000000, -5.250000000000000000 ) ) ;
#9029=CARTESIAN_POINT ( 'NONE',  ( -1.084901341431563923E-15, -27.73437500034139802, 5.905927827173866440 ) ) ;
#9034=CARTESIAN_POINT ( 'NONE',  ( 5.114683531250000748, -29.42187500034139802, 0.000000000000000000 ) ) ;
#9035=CARTESIAN_POINT ( 'NONE',  ( -5.250000000000000000, -28.37499999999999645, -6.429395695523604153E-16 ) ) ;
#9036=CARTESIAN_POINT ( 'NONE',  ( 5.114683531249999859, -29.15104166700806232, -2.952963913586932776 ) ) ;
#9037=CARTESIAN_POINT ( 'NONE',  ( -2.624999999999998668, -28.44791666734946389, -4.546633369868303021 ) ) ;
#9040=CARTESIAN_POINT ( 'NONE',  ( 6.429395695523604153E-16, -30.00000000000000000, -5.250000000000000000 ) ) ;
#9046=CARTESIAN_POINT ( 'NONE',  ( 2.625000000000000444, -27.73958333401612819, -4.546633369868303021 ) ) ;
#9048=ORIENTED_EDGE ( 'NONE', *, *, #8523, .T. ) ;
#9052=CARTESIAN_POINT ( 'NONE',  ( 1.406733260263391960, -29.55133545031537068, 5.250000000000000000 ) ) ;
#9056=CIRCLE ( 'NONE', #136, 4.250000000000000000 ) ;
#9057=CARTESIAN_POINT ( 'NONE',  ( 5.249999999999997335, -28.05208333401612819, 3.031088913245538308 ) ) ;
#9058=CARTESIAN_POINT ( 'NONE',  ( 2.557341765625000818, -28.06770833367473017, -4.429445870380400052 ) ) ;
#9064=EDGE_CURVE ( 'NONE', #8178, #627, #2060, .T. ) ;
#9068=CARTESIAN_POINT ( 'NONE',  ( 5.250000000000000000, -28.99999999999999645, 0.000000000000000000 ) ) ;
#9070=DIRECTION ( 'NONE',  ( 0.000000000000000000, 1.000000000000000000, 0.000000000000000000 ) ) ;
#9071=ORIENTED_EDGE ( 'NONE', *, *, #3103, .T. ) ;
#9075=CARTESIAN_POINT ( 'NONE',  ( 2.557341765624996821, -27.40104166700806587, 4.429445870380401828 ) ) ;
#9077=CARTESIAN_POINT ( 'NONE',  ( -5.250000000000000888, -29.85416666666666785, 3.031088913245532979 ) ) ;
#9079=( BOUNDED_CURVE ( )  B_SPLINE_CURVE ( 2, ( #416, #4745, #8926, #5487, #4834, #7680, #6145, #4057, #4791 ),
 .UNSPECIFIED., .F., .T. ) 
 B_SPLINE_CURVE_WITH_KNOTS ( ( 3, 2, 2, 2, 3 ),
 ( 0.8541666666666666297, 0.8611111111111111605, 0.8750000000000000000, 0.8888888888888888395, 0.8958333333333333703 ),
 .UNSPECIFIED. ) 
 CURVE ( )  GEOMETRIC_REPRESENTATION_ITEM ( )  RATIONAL_B_SPLINE_CURVE ( ( 0.9330127018922192983, 0.9330127018922187432, 1.000000000000000000, 0.8660254037844387076, 1.000000000000000000, 0.8660254037844387076, 1.000000000000000000, 0.9330127018922187432, 0.9330127018922192983 ) ) 
 REPRESENTATION_ITEM ( '' )  );
#9080=CARTESIAN_POINT ( 'NONE',  ( 3.616337804771879580E-16, -29.35937500034139802, -5.905927827173866440 ) ) ;
#9081=DIRECTION ( 'NONE',  ( 0.000000000000000000, 0.000000000000000000, 1.000000000000000000 ) ) ;
#9082=CARTESIAN_POINT ( 'NONE',  ( 2.557341765625000818, -29.13020833367473017, -4.429445870380400052 ) ) ;
#9086=CARTESIAN_POINT ( 'NONE',  ( 5.250000000000000000, -29.53125000068279604, 0.000000000000000000 ) ) ;
#9092=CARTESIAN_POINT ( 'NONE',  ( 5.250000000000000000, -26.78125000068279604, 0.000000000000000000 ) ) ;
#9097=CARTESIAN_POINT ( 'NONE',  ( 2.033577675846918216E-14, -27.06250000000000355, 5.250000000000000888 ) ) ;
#9098=EDGE_CURVE ( 'NONE', #5221, #7067, #7993, .T. ) ;
#9103=CARTESIAN_POINT ( 'NONE',  ( -2.557341765625002594, -29.19270833367473017, 4.429445870380399164 ) ) ;
#9105=PRODUCT_DEFINITION ( 'UNKNOWN', '', #1755, #3017 ) ;
#9112=AXIS2_PLACEMENT_3D ( 'NONE', #6758, #2675, #1227 ) ;
#9113=LINE ( 'NONE', #7591, #5395 ) ;
#9114=CARTESIAN_POINT ( 'NONE',  ( 0.000000000000000000, -9.999999999999998224, 5.750000000000000000 ) ) ;
#9119=CARTESIAN_POINT ( 'NONE',  ( 5.114683531250000748, -27.08854166700806232, -2.952963913586932776 ) ) ;
#9121=CARTESIAN_POINT ( 'NONE',  ( -5.114683531249999859, -27.81770833367473017, -2.952963913586935440 ) ) ;
#9123=CARTESIAN_POINT ( 'NONE',  ( 3.616337804771879580E-16, -29.10937500034139802, -5.905927827173866440 ) ) ;
#9126=CARTESIAN_POINT ( 'NONE',  ( 5.114683531249998971, -29.44270833367473372, 2.952963913586936329 ) ) ;
#9130=CARTESIAN_POINT ( 'NONE',  ( -1.975475456537005874E-15, -29.59375000068279249, 5.250000000000000000 ) ) ;
#9135=ORIENTED_EDGE ( 'NONE', *, *, #74, .T. ) ;
#9137=CARTESIAN_POINT ( 'NONE',  ( -5.250000000000000000, -26.90625000068279604, -6.429395695523604153E-16 ) ) ;
#9140=ADVANCED_FACE ( 'NONE', ( #8258 ), #7605, .F. ) ;
#9144=CARTESIAN_POINT ( 'NONE',  ( 5.250000000000000000, -26.78125000068279604, 0.000000000000000000 ) ) ;
#9146=CARTESIAN_POINT ( 'NONE',  ( -2.557341765624999042, -28.27604166700806587, -4.429445870380400052 ) ) ;
#9148=CARTESIAN_POINT ( 'NONE',  ( -1.406733260263395735, -28.85491455036742892, 5.250000000000000000 ) ) ;
#9153=CARTESIAN_POINT ( 'NONE',  ( 0.000000000000000000, -30.00000000000000000, 5.250000000000000000 ) ) ;
#9157=ORIENTED_EDGE ( 'NONE', *, *, #6457, .T. ) ;
#9158=CARTESIAN_POINT ( 'NONE',  ( -1.084901341431563726E-15, -27.92187500034139802, 5.905927827173866440 ) ) ;
#9160=CARTESIAN_POINT ( 'NONE',  ( 5.250000000000000000, -29.47916666666666430, -3.031088913245534755 ) ) ;
#9161=DIRECTION ( 'NONE',  ( 0.000000000000000000, 0.000000000000000000, 1.000000000000000000 ) ) ;
#9164=CARTESIAN_POINT ( 'NONE',  ( 5.114683531250000748, -29.65104166700806232, -2.952963913586932776 ) ) ;
#9165=CARTESIAN_POINT ( 'NONE',  ( -1.084901341431563923E-15, -27.73437500034139802, 5.905927827173866440 ) ) ;
#9174=ORIENTED_EDGE ( 'NONE', *, *, #4012, .T. ) ;
#9176=CARTESIAN_POINT ( 'NONE',  ( -5.114683531250000748, -29.73437500034139802, -6.263680815196995234E-16 ) ) ;
#9181=CIRCLE ( 'NONE', #575, 4.250000000000000000 ) ;
#9182=ORIENTED_EDGE ( 'NONE', *, *, #7525, .T. ) ;
#9186=AXIS2_PLACEMENT_3D ( 'NONE', #356, #3208, #1289 ) ;
#9187=CARTESIAN_POINT ( 'NONE',  ( -1.084901341431563923E-15, -28.92187500034139447, 5.905927827173866440 ) ) ;
#9198=COLOUR_RGB('Dark Blue',0.08,0.2,0.34);
#9199=FILL_AREA_STYLE_COLOUR('',#9198);
#9200=FILL_AREA_STYLE('',(#9199));
#9201=SURFACE_STYLE_FILL_AREA(#9200);
#9202=SURFACE_SIDE_STYLE('',(#9201));
#9203=SURFACE_STYLE_USAGE(.BOTH.,#9202);
#9204=PRESENTATION_STYLE_ASSIGNMENT((#9203));
ENDSEC;
END-ISO-10303-21;
